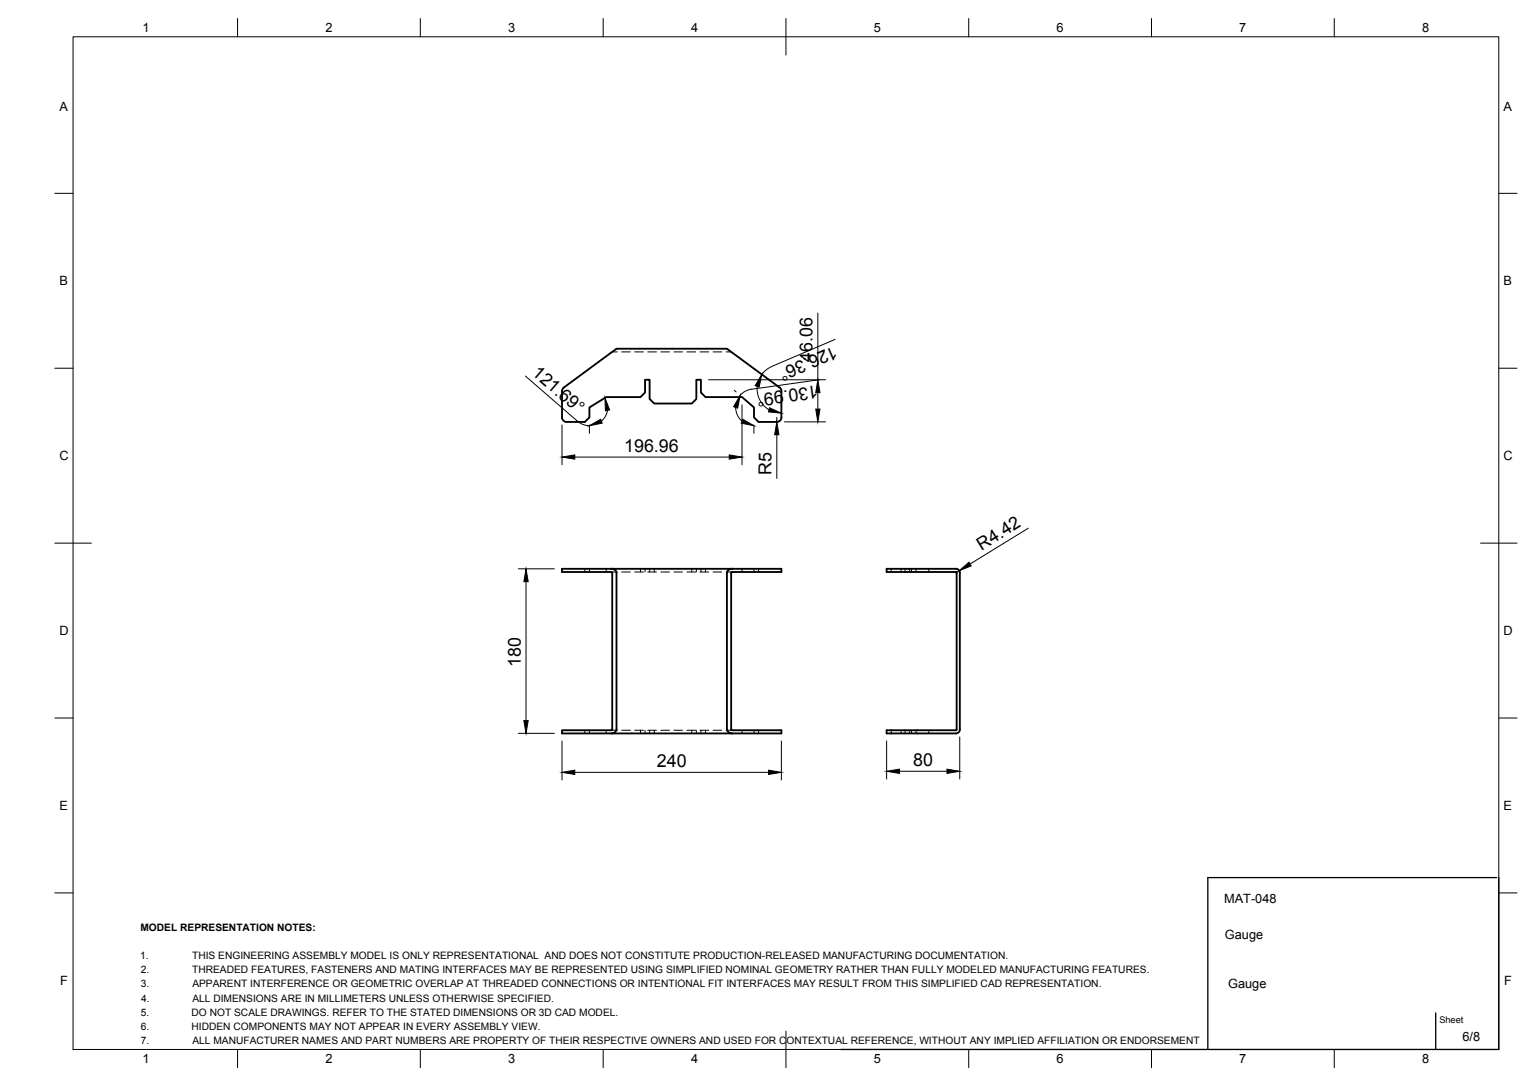
ISO-10303-21;
HEADER;
/* Generated by software containing ST-Developer
 * from STEP Tools, Inc. (www.steptools.com) 
 */

FILE_DESCRIPTION(
/* description */ ('STEP AP214'),
/* implementation_level */ '2;1');

FILE_NAME(
/* name */ 'Gauge.step',
/* time_stamp */ '2026-11-14T22:24:45-08:00',
/* author */ (''),
/* organization */ (''),
/* preprocessor_version */ 'ST-DEVELOPER v20.2',
/* originating_system */ 'Autodesk Translation Framework v15.17.0.0',
/* authorisation */ '');

FILE_SCHEMA (('AUTOMOTIVE_DESIGN { 1 0 10303 214 3 1 1 }'));
ENDSEC;

DATA;
#10=MECHANICAL_DESIGN_GEOMETRIC_PRESENTATION_REPRESENTATION('',(#125),#5599);
#113=SHAPE_REPRESENTATION_RELATIONSHIP('SRR','None',#5641,#119);
#119=ADVANCED_BREP_SHAPE_REPRESENTATION('',(#131),#5593);
#125=STYLED_ITEM('',(#5680),#131);
#131=MANIFOLD_SOLID_BREP('Body1',#3307);
#137=ELLIPSE('',#3398,7.45592114551632,4.41999999999987);
#138=ELLIPSE('',#3399,7.45592114551703,4.42000000000052);
#139=ELLIPSE('',#3402,7.45592114551723,4.42000000000049);
#140=ELLIPSE('',#3403,7.45592114551628,4.41999999999988);
#141=ELLIPSE('',#3416,1.68685998767419,1.00000000000061);
#142=ELLIPSE('',#3417,1.68685998767298,0.999999999999771);
#143=ELLIPSE('',#3420,1.68685998767017,0.999999999998458);
#144=ELLIPSE('',#3421,1.68685998767381,1.0000000000002);
#145=CYLINDRICAL_SURFACE('',#3397,4.42000000000001);
#146=CYLINDRICAL_SURFACE('',#3401,4.42);
#147=CYLINDRICAL_SURFACE('',#3415,1.);
#148=CYLINDRICAL_SURFACE('',#3419,1.);
#149=CYLINDRICAL_SURFACE('',#3464,5.);
#150=CYLINDRICAL_SURFACE('',#3465,5.);
#151=CYLINDRICAL_SURFACE('',#3466,5.);
#152=CYLINDRICAL_SURFACE('',#3467,5.);
#153=CYLINDRICAL_SURFACE('',#3468,5.);
#154=CYLINDRICAL_SURFACE('',#3469,5.);
#155=CYLINDRICAL_SURFACE('',#3470,5.);
#156=CYLINDRICAL_SURFACE('',#3471,5.);
#193=CIRCLE('',#3387,5.);
#194=CIRCLE('',#3388,5.);
#195=CIRCLE('',#3389,5.);
#196=CIRCLE('',#3390,5.);
#197=CIRCLE('',#3393,5.);
#198=CIRCLE('',#3394,5.);
#199=CIRCLE('',#3395,5.);
#200=CIRCLE('',#3396,5.);
#201=CIRCLE('',#3405,5.);
#202=CIRCLE('',#3406,5.);
#203=CIRCLE('',#3407,5.);
#204=CIRCLE('',#3408,5.);
#205=CIRCLE('',#3411,5.);
#206=CIRCLE('',#3412,5.);
#207=CIRCLE('',#3413,5.);
#208=CIRCLE('',#3414,5.);
#281=FACE_OUTER_BOUND('',#457,.T.);
#282=FACE_OUTER_BOUND('',#458,.T.);
#283=FACE_OUTER_BOUND('',#459,.T.);
#284=FACE_OUTER_BOUND('',#460,.T.);
#285=FACE_OUTER_BOUND('',#461,.T.);
#286=FACE_OUTER_BOUND('',#462,.T.);
#287=FACE_OUTER_BOUND('',#463,.T.);
#288=FACE_OUTER_BOUND('',#464,.T.);
#289=FACE_OUTER_BOUND('',#465,.T.);
#290=FACE_OUTER_BOUND('',#466,.T.);
#291=FACE_OUTER_BOUND('',#467,.T.);
#292=FACE_OUTER_BOUND('',#468,.T.);
#293=FACE_OUTER_BOUND('',#469,.T.);
#294=FACE_OUTER_BOUND('',#470,.T.);
#295=FACE_OUTER_BOUND('',#471,.T.);
#296=FACE_OUTER_BOUND('',#472,.T.);
#297=FACE_OUTER_BOUND('',#473,.T.);
#298=FACE_OUTER_BOUND('',#474,.T.);
#299=FACE_OUTER_BOUND('',#475,.T.);
#300=FACE_OUTER_BOUND('',#476,.T.);
#301=FACE_OUTER_BOUND('',#477,.T.);
#302=FACE_OUTER_BOUND('',#478,.T.);
#303=FACE_OUTER_BOUND('',#479,.T.);
#304=FACE_OUTER_BOUND('',#480,.T.);
#305=FACE_OUTER_BOUND('',#481,.T.);
#306=FACE_OUTER_BOUND('',#482,.T.);
#307=FACE_OUTER_BOUND('',#483,.T.);
#308=FACE_OUTER_BOUND('',#484,.T.);
#309=FACE_OUTER_BOUND('',#485,.T.);
#310=FACE_OUTER_BOUND('',#486,.T.);
#311=FACE_OUTER_BOUND('',#487,.T.);
#312=FACE_OUTER_BOUND('',#488,.T.);
#313=FACE_OUTER_BOUND('',#489,.T.);
#314=FACE_OUTER_BOUND('',#490,.T.);
#315=FACE_OUTER_BOUND('',#491,.T.);
#316=FACE_OUTER_BOUND('',#492,.T.);
#317=FACE_OUTER_BOUND('',#493,.T.);
#318=FACE_OUTER_BOUND('',#494,.T.);
#319=FACE_OUTER_BOUND('',#495,.T.);
#320=FACE_OUTER_BOUND('',#496,.T.);
#321=FACE_OUTER_BOUND('',#497,.T.);
#322=FACE_OUTER_BOUND('',#498,.T.);
#323=FACE_OUTER_BOUND('',#499,.T.);
#324=FACE_OUTER_BOUND('',#500,.T.);
#325=FACE_OUTER_BOUND('',#501,.T.);
#326=FACE_OUTER_BOUND('',#502,.T.);
#327=FACE_OUTER_BOUND('',#503,.T.);
#328=FACE_OUTER_BOUND('',#504,.T.);
#329=FACE_OUTER_BOUND('',#505,.T.);
#330=FACE_OUTER_BOUND('',#506,.T.);
#331=FACE_OUTER_BOUND('',#507,.T.);
#332=FACE_OUTER_BOUND('',#508,.T.);
#333=FACE_OUTER_BOUND('',#509,.T.);
#334=FACE_OUTER_BOUND('',#510,.T.);
#335=FACE_OUTER_BOUND('',#511,.T.);
#336=FACE_OUTER_BOUND('',#512,.T.);
#337=FACE_OUTER_BOUND('',#513,.T.);
#338=FACE_OUTER_BOUND('',#514,.T.);
#339=FACE_OUTER_BOUND('',#515,.T.);
#340=FACE_OUTER_BOUND('',#516,.T.);
#341=FACE_OUTER_BOUND('',#517,.T.);
#342=FACE_OUTER_BOUND('',#518,.T.);
#343=FACE_OUTER_BOUND('',#519,.T.);
#344=FACE_OUTER_BOUND('',#520,.T.);
#345=FACE_OUTER_BOUND('',#521,.T.);
#346=FACE_OUTER_BOUND('',#522,.T.);
#457=EDGE_LOOP('',(#2099,#2100,#2101,#2102));
#458=EDGE_LOOP('',(#2103,#2104,#2105,#2106));
#459=EDGE_LOOP('',(#2107,#2108,#2109,#2110));
#460=EDGE_LOOP('',(#2111,#2112,#2113,#2114));
#461=EDGE_LOOP('',(#2115,#2116,#2117,#2118,#2119,#2120,#2121,#2122,#2123,
#2124,#2125,#2126,#2127,#2128,#2129,#2130,#2131,#2132,#2133,#2134,#2135,
#2136,#2137,#2138,#2139,#2140,#2141,#2142,#2143,#2144));
#462=EDGE_LOOP('',(#2145,#2146,#2147,#2148));
#463=EDGE_LOOP('',(#2149,#2150,#2151,#2152,#2153,#2154,#2155,#2156,#2157,
#2158,#2159,#2160,#2161,#2162,#2163,#2164,#2165,#2166,#2167,#2168,#2169,
#2170,#2171,#2172,#2173,#2174,#2175,#2176,#2177,#2178));
#464=EDGE_LOOP('',(#2179,#2180,#2181,#2182));
#465=EDGE_LOOP('',(#2183,#2184,#2185,#2186));
#466=EDGE_LOOP('',(#2187,#2188,#2189,#2190));
#467=EDGE_LOOP('',(#2191,#2192,#2193,#2194,#2195,#2196,#2197,#2198,#2199,
#2200,#2201,#2202,#2203,#2204,#2205,#2206,#2207,#2208,#2209,#2210,#2211,
#2212,#2213,#2214,#2215,#2216,#2217,#2218,#2219,#2220));
#468=EDGE_LOOP('',(#2221,#2222,#2223,#2224));
#469=EDGE_LOOP('',(#2225,#2226,#2227,#2228,#2229,#2230,#2231,#2232,#2233,
#2234,#2235,#2236,#2237,#2238,#2239,#2240,#2241,#2242,#2243,#2244,#2245,
#2246,#2247,#2248,#2249,#2250,#2251,#2252,#2253,#2254));
#470=EDGE_LOOP('',(#2255,#2256,#2257,#2258));
#471=EDGE_LOOP('',(#2259,#2260,#2261,#2262));
#472=EDGE_LOOP('',(#2263,#2264,#2265,#2266));
#473=EDGE_LOOP('',(#2267,#2268,#2269,#2270));
#474=EDGE_LOOP('',(#2271,#2272,#2273,#2274));
#475=EDGE_LOOP('',(#2275,#2276,#2277,#2278,#2279,#2280,#2281,#2282,#2283,
#2284,#2285,#2286));
#476=EDGE_LOOP('',(#2287,#2288,#2289,#2290,#2291,#2292,#2293,#2294,#2295,
#2296,#2297,#2298));
#477=EDGE_LOOP('',(#2299,#2300,#2301,#2302));
#478=EDGE_LOOP('',(#2303,#2304,#2305,#2306));
#479=EDGE_LOOP('',(#2307,#2308,#2309,#2310));
#480=EDGE_LOOP('',(#2311,#2312,#2313,#2314));
#481=EDGE_LOOP('',(#2315,#2316,#2317,#2318));
#482=EDGE_LOOP('',(#2319,#2320,#2321,#2322));
#483=EDGE_LOOP('',(#2323,#2324,#2325,#2326));
#484=EDGE_LOOP('',(#2327,#2328,#2329,#2330));
#485=EDGE_LOOP('',(#2331,#2332,#2333,#2334));
#486=EDGE_LOOP('',(#2335,#2336,#2337,#2338));
#487=EDGE_LOOP('',(#2339,#2340,#2341,#2342));
#488=EDGE_LOOP('',(#2343,#2344,#2345,#2346));
#489=EDGE_LOOP('',(#2347,#2348,#2349,#2350));
#490=EDGE_LOOP('',(#2351,#2352,#2353,#2354));
#491=EDGE_LOOP('',(#2355,#2356,#2357,#2358));
#492=EDGE_LOOP('',(#2359,#2360,#2361,#2362));
#493=EDGE_LOOP('',(#2363,#2364,#2365,#2366));
#494=EDGE_LOOP('',(#2367,#2368,#2369,#2370));
#495=EDGE_LOOP('',(#2371,#2372,#2373,#2374));
#496=EDGE_LOOP('',(#2375,#2376,#2377,#2378));
#497=EDGE_LOOP('',(#2379,#2380,#2381,#2382));
#498=EDGE_LOOP('',(#2383,#2384,#2385,#2386));
#499=EDGE_LOOP('',(#2387,#2388,#2389,#2390));
#500=EDGE_LOOP('',(#2391,#2392,#2393,#2394));
#501=EDGE_LOOP('',(#2395,#2396,#2397,#2398));
#502=EDGE_LOOP('',(#2399,#2400,#2401,#2402));
#503=EDGE_LOOP('',(#2403,#2404,#2405,#2406));
#504=EDGE_LOOP('',(#2407,#2408,#2409,#2410));
#505=EDGE_LOOP('',(#2411,#2412,#2413,#2414));
#506=EDGE_LOOP('',(#2415,#2416,#2417,#2418));
#507=EDGE_LOOP('',(#2419,#2420,#2421,#2422));
#508=EDGE_LOOP('',(#2423,#2424,#2425,#2426));
#509=EDGE_LOOP('',(#2427,#2428,#2429,#2430));
#510=EDGE_LOOP('',(#2431,#2432,#2433,#2434));
#511=EDGE_LOOP('',(#2435,#2436,#2437,#2438));
#512=EDGE_LOOP('',(#2439,#2440,#2441,#2442));
#513=EDGE_LOOP('',(#2443,#2444,#2445,#2446));
#514=EDGE_LOOP('',(#2447,#2448,#2449,#2450));
#515=EDGE_LOOP('',(#2451,#2452,#2453,#2454));
#516=EDGE_LOOP('',(#2455,#2456,#2457,#2458));
#517=EDGE_LOOP('',(#2459,#2460,#2461,#2462));
#518=EDGE_LOOP('',(#2463,#2464,#2465,#2466));
#519=EDGE_LOOP('',(#2467,#2468,#2469,#2470));
#520=EDGE_LOOP('',(#2471,#2472,#2473,#2474));
#521=EDGE_LOOP('',(#2475,#2476,#2477,#2478));
#522=EDGE_LOOP('',(#2479,#2480,#2481,#2482));
#647=LINE('',#4644,#1003);
#648=LINE('',#4646,#1004);
#649=LINE('',#4648,#1005);
#650=LINE('',#4649,#1006);
#651=LINE('',#4653,#1007);
#652=LINE('',#4655,#1008);
#653=LINE('',#4657,#1009);
#654=LINE('',#4658,#1010);
#655=LINE('',#4662,#1011);
#656=LINE('',#4664,#1012);
#657=LINE('',#4666,#1013);
#658=LINE('',#4667,#1014);
#659=LINE('',#4671,#1015);
#660=LINE('',#4673,#1016);
#661=LINE('',#4675,#1017);
#662=LINE('',#4676,#1018);
#663=LINE('',#4680,#1019);
#664=LINE('',#4684,#1020);
#665=LINE('',#4686,#1021);
#666=LINE('',#4688,#1022);
#667=LINE('',#4690,#1023);
#668=LINE('',#4692,#1024);
#669=LINE('',#4694,#1025);
#670=LINE('',#4696,#1026);
#671=LINE('',#4698,#1027);
#672=LINE('',#4700,#1028);
#673=LINE('',#4702,#1029);
#674=LINE('',#4704,#1030);
#675=LINE('',#4706,#1031);
#676=LINE('',#4708,#1032);
#677=LINE('',#4710,#1033);
#678=LINE('',#4712,#1034);
#679=LINE('',#4714,#1035);
#680=LINE('',#4716,#1036);
#681=LINE('',#4718,#1037);
#682=LINE('',#4720,#1038);
#683=LINE('',#4721,#1039);
#684=LINE('',#4726,#1040);
#685=LINE('',#4728,#1041);
#686=LINE('',#4730,#1042);
#687=LINE('',#4734,#1043);
#688=LINE('',#4736,#1044);
#689=LINE('',#4737,#1045);
#690=LINE('',#4742,#1046);
#691=LINE('',#4746,#1047);
#692=LINE('',#4748,#1048);
#693=LINE('',#4750,#1049);
#694=LINE('',#4754,#1050);
#695=LINE('',#4756,#1051);
#696=LINE('',#4758,#1052);
#697=LINE('',#4760,#1053);
#698=LINE('',#4762,#1054);
#699=LINE('',#4764,#1055);
#700=LINE('',#4766,#1056);
#701=LINE('',#4768,#1057);
#702=LINE('',#4770,#1058);
#703=LINE('',#4772,#1059);
#704=LINE('',#4774,#1060);
#705=LINE('',#4776,#1061);
#706=LINE('',#4778,#1062);
#707=LINE('',#4780,#1063);
#708=LINE('',#4782,#1064);
#709=LINE('',#4784,#1065);
#710=LINE('',#4786,#1066);
#711=LINE('',#4788,#1067);
#712=LINE('',#4789,#1068);
#713=LINE('',#4795,#1069);
#714=LINE('',#4798,#1070);
#715=LINE('',#4800,#1071);
#716=LINE('',#4801,#1072);
#717=LINE('',#4807,#1073);
#718=LINE('',#4812,#1074);
#719=LINE('',#4814,#1075);
#720=LINE('',#4816,#1076);
#721=LINE('',#4818,#1077);
#722=LINE('',#4820,#1078);
#723=LINE('',#4822,#1079);
#724=LINE('',#4824,#1080);
#725=LINE('',#4826,#1081);
#726=LINE('',#4828,#1082);
#727=LINE('',#4830,#1083);
#728=LINE('',#4832,#1084);
#729=LINE('',#4834,#1085);
#730=LINE('',#4836,#1086);
#731=LINE('',#4838,#1087);
#732=LINE('',#4840,#1088);
#733=LINE('',#4842,#1089);
#734=LINE('',#4844,#1090);
#735=LINE('',#4846,#1091);
#736=LINE('',#4848,#1092);
#737=LINE('',#4849,#1093);
#738=LINE('',#4853,#1094);
#739=LINE('',#4856,#1095);
#740=LINE('',#4858,#1096);
#741=LINE('',#4862,#1097);
#742=LINE('',#4864,#1098);
#743=LINE('',#4865,#1099);
#744=LINE('',#4871,#1100);
#745=LINE('',#4873,#1101);
#746=LINE('',#4875,#1102);
#747=LINE('',#4879,#1103);
#748=LINE('',#4882,#1104);
#749=LINE('',#4884,#1105);
#750=LINE('',#4886,#1106);
#751=LINE('',#4888,#1107);
#752=LINE('',#4890,#1108);
#753=LINE('',#4892,#1109);
#754=LINE('',#4894,#1110);
#755=LINE('',#4896,#1111);
#756=LINE('',#4898,#1112);
#757=LINE('',#4900,#1113);
#758=LINE('',#4902,#1114);
#759=LINE('',#4904,#1115);
#760=LINE('',#4906,#1116);
#761=LINE('',#4908,#1117);
#762=LINE('',#4910,#1118);
#763=LINE('',#4912,#1119);
#764=LINE('',#4914,#1120);
#765=LINE('',#4916,#1121);
#766=LINE('',#4917,#1122);
#767=LINE('',#4921,#1123);
#768=LINE('',#4927,#1124);
#769=LINE('',#4928,#1125);
#770=LINE('',#4929,#1126);
#771=LINE('',#4934,#1127);
#772=LINE('',#4935,#1128);
#773=LINE('',#4937,#1129);
#774=LINE('',#4938,#1130);
#775=LINE('',#4940,#1131);
#776=LINE('',#4941,#1132);
#777=LINE('',#4943,#1133);
#778=LINE('',#4944,#1134);
#779=LINE('',#4946,#1135);
#780=LINE('',#4947,#1136);
#781=LINE('',#4949,#1137);
#782=LINE('',#4950,#1138);
#783=LINE('',#4952,#1139);
#784=LINE('',#4954,#1140);
#785=LINE('',#4956,#1141);
#786=LINE('',#4957,#1142);
#787=LINE('',#4959,#1143);
#788=LINE('',#4961,#1144);
#789=LINE('',#4963,#1145);
#790=LINE('',#4964,#1146);
#791=LINE('',#4966,#1147);
#792=LINE('',#4967,#1148);
#793=LINE('',#4969,#1149);
#794=LINE('',#4971,#1150);
#795=LINE('',#4973,#1151);
#796=LINE('',#4974,#1152);
#797=LINE('',#4977,#1153);
#798=LINE('',#4978,#1154);
#799=LINE('',#4980,#1155);
#800=LINE('',#4982,#1156);
#801=LINE('',#4983,#1157);
#802=LINE('',#4985,#1158);
#803=LINE('',#4987,#1159);
#804=LINE('',#4989,#1160);
#805=LINE('',#4990,#1161);
#806=LINE('',#4992,#1162);
#807=LINE('',#4993,#1163);
#808=LINE('',#4995,#1164);
#809=LINE('',#4997,#1165);
#810=LINE('',#4999,#1166);
#811=LINE('',#5000,#1167);
#812=LINE('',#5002,#1168);
#813=LINE('',#5004,#1169);
#814=LINE('',#5006,#1170);
#1003=VECTOR('',#3687,1000.);
#1004=VECTOR('',#3688,1000.);
#1005=VECTOR('',#3689,1000.);
#1006=VECTOR('',#3690,1000.);
#1007=VECTOR('',#3693,1000.);
#1008=VECTOR('',#3694,1000.);
#1009=VECTOR('',#3695,1000.);
#1010=VECTOR('',#3696,1000.);
#1011=VECTOR('',#3699,1000.);
#1012=VECTOR('',#3700,1000.);
#1013=VECTOR('',#3701,1000.);
#1014=VECTOR('',#3702,1000.);
#1015=VECTOR('',#3705,1000.);
#1016=VECTOR('',#3706,1000.);
#1017=VECTOR('',#3707,1000.);
#1018=VECTOR('',#3708,1000.);
#1019=VECTOR('',#3711,1000.);
#1020=VECTOR('',#3714,1000.);
#1021=VECTOR('',#3715,1000.);
#1022=VECTOR('',#3716,1000.);
#1023=VECTOR('',#3717,1000.);
#1024=VECTOR('',#3718,1000.);
#1025=VECTOR('',#3719,1000.);
#1026=VECTOR('',#3720,1000.);
#1027=VECTOR('',#3721,1000.);
#1028=VECTOR('',#3722,1000.);
#1029=VECTOR('',#3723,1000.);
#1030=VECTOR('',#3724,1000.);
#1031=VECTOR('',#3725,1000.);
#1032=VECTOR('',#3726,1000.);
#1033=VECTOR('',#3727,1000.);
#1034=VECTOR('',#3728,1000.);
#1035=VECTOR('',#3729,1000.);
#1036=VECTOR('',#3730,1000.);
#1037=VECTOR('',#3731,1000.);
#1038=VECTOR('',#3732,1000.);
#1039=VECTOR('',#3733,1000.);
#1040=VECTOR('',#3738,1000.);
#1041=VECTOR('',#3739,1000.);
#1042=VECTOR('',#3740,1000.);
#1043=VECTOR('',#3745,1000.);
#1044=VECTOR('',#3746,1000.);
#1045=VECTOR('',#3747,1000.);
#1046=VECTOR('',#3752,1000.);
#1047=VECTOR('',#3755,1000.);
#1048=VECTOR('',#3756,1000.);
#1049=VECTOR('',#3757,1000.);
#1050=VECTOR('',#3762,1000.);
#1051=VECTOR('',#3763,1000.);
#1052=VECTOR('',#3764,1000.);
#1053=VECTOR('',#3765,1000.);
#1054=VECTOR('',#3766,1000.);
#1055=VECTOR('',#3767,1000.);
#1056=VECTOR('',#3768,1000.);
#1057=VECTOR('',#3769,1000.);
#1058=VECTOR('',#3770,1000.);
#1059=VECTOR('',#3771,1000.);
#1060=VECTOR('',#3772,1000.);
#1061=VECTOR('',#3773,1000.);
#1062=VECTOR('',#3774,1000.);
#1063=VECTOR('',#3775,1000.);
#1064=VECTOR('',#3776,1000.);
#1065=VECTOR('',#3777,1000.);
#1066=VECTOR('',#3778,1000.);
#1067=VECTOR('',#3779,1000.);
#1068=VECTOR('',#3780,1000.);
#1069=VECTOR('',#3787,1000.);
#1070=VECTOR('',#3790,1000.);
#1071=VECTOR('',#3791,1000.);
#1072=VECTOR('',#3792,1000.);
#1073=VECTOR('',#3799,1000.);
#1074=VECTOR('',#3804,1000.);
#1075=VECTOR('',#3805,1000.);
#1076=VECTOR('',#3806,1000.);
#1077=VECTOR('',#3807,1000.);
#1078=VECTOR('',#3808,1000.);
#1079=VECTOR('',#3809,1000.);
#1080=VECTOR('',#3810,1000.);
#1081=VECTOR('',#3811,1000.);
#1082=VECTOR('',#3812,1000.);
#1083=VECTOR('',#3813,1000.);
#1084=VECTOR('',#3814,1000.);
#1085=VECTOR('',#3815,1000.);
#1086=VECTOR('',#3816,1000.);
#1087=VECTOR('',#3817,1000.);
#1088=VECTOR('',#3818,1000.);
#1089=VECTOR('',#3819,1000.);
#1090=VECTOR('',#3820,1000.);
#1091=VECTOR('',#3821,1000.);
#1092=VECTOR('',#3822,1000.);
#1093=VECTOR('',#3823,1000.);
#1094=VECTOR('',#3826,1000.);
#1095=VECTOR('',#3829,1000.);
#1096=VECTOR('',#3830,1000.);
#1097=VECTOR('',#3835,1000.);
#1098=VECTOR('',#3836,1000.);
#1099=VECTOR('',#3837,1000.);
#1100=VECTOR('',#3844,1000.);
#1101=VECTOR('',#3845,1000.);
#1102=VECTOR('',#3846,1000.);
#1103=VECTOR('',#3849,1000.);
#1104=VECTOR('',#3852,1000.);
#1105=VECTOR('',#3853,1000.);
#1106=VECTOR('',#3854,1000.);
#1107=VECTOR('',#3855,1000.);
#1108=VECTOR('',#3856,1000.);
#1109=VECTOR('',#3857,1000.);
#1110=VECTOR('',#3858,1000.);
#1111=VECTOR('',#3859,1000.);
#1112=VECTOR('',#3860,1000.);
#1113=VECTOR('',#3861,1000.);
#1114=VECTOR('',#3862,1000.);
#1115=VECTOR('',#3863,1000.);
#1116=VECTOR('',#3864,1000.);
#1117=VECTOR('',#3865,1000.);
#1118=VECTOR('',#3866,1000.);
#1119=VECTOR('',#3867,1000.);
#1120=VECTOR('',#3868,1000.);
#1121=VECTOR('',#3869,1000.);
#1122=VECTOR('',#3870,1000.);
#1123=VECTOR('',#3873,1000.);
#1124=VECTOR('',#3880,1000.);
#1125=VECTOR('',#3881,1000.);
#1126=VECTOR('',#3882,1000.);
#1127=VECTOR('',#3891,1000.);
#1128=VECTOR('',#3892,1000.);
#1129=VECTOR('',#3895,1000.);
#1130=VECTOR('',#3896,1000.);
#1131=VECTOR('',#3899,1000.);
#1132=VECTOR('',#3900,1000.);
#1133=VECTOR('',#3903,1000.);
#1134=VECTOR('',#3904,1000.);
#1135=VECTOR('',#3907,1000.);
#1136=VECTOR('',#3908,1000.);
#1137=VECTOR('',#3911,1000.);
#1138=VECTOR('',#3912,1000.);
#1139=VECTOR('',#3915,1000.);
#1140=VECTOR('',#3918,1000.);
#1141=VECTOR('',#3921,1000.);
#1142=VECTOR('',#3922,1000.);
#1143=VECTOR('',#3925,1000.);
#1144=VECTOR('',#3928,1000.);
#1145=VECTOR('',#3931,1000.);
#1146=VECTOR('',#3932,1000.);
#1147=VECTOR('',#3935,1000.);
#1148=VECTOR('',#3936,1000.);
#1149=VECTOR('',#3939,1000.);
#1150=VECTOR('',#3942,1000.);
#1151=VECTOR('',#3945,1000.);
#1152=VECTOR('',#3946,1000.);
#1153=VECTOR('',#3951,1000.);
#1154=VECTOR('',#3952,1000.);
#1155=VECTOR('',#3955,1000.);
#1156=VECTOR('',#3958,1000.);
#1157=VECTOR('',#3959,1000.);
#1158=VECTOR('',#3962,1000.);
#1159=VECTOR('',#3965,1000.);
#1160=VECTOR('',#3968,1000.);
#1161=VECTOR('',#3969,1000.);
#1162=VECTOR('',#3972,1000.);
#1163=VECTOR('',#3973,1000.);
#1164=VECTOR('',#3976,1000.);
#1165=VECTOR('',#3979,1000.);
#1166=VECTOR('',#3982,1000.);
#1167=VECTOR('',#3983,1000.);
#1168=VECTOR('',#3986,1000.);
#1169=VECTOR('',#3989,1000.);
#1170=VECTOR('',#3992,1000.);
#1359=VERTEX_POINT('',#4642);
#1360=VERTEX_POINT('',#4643);
#1361=VERTEX_POINT('',#4645);
#1362=VERTEX_POINT('',#4647);
#1363=VERTEX_POINT('',#4651);
#1364=VERTEX_POINT('',#4652);
#1365=VERTEX_POINT('',#4654);
#1366=VERTEX_POINT('',#4656);
#1367=VERTEX_POINT('',#4660);
#1368=VERTEX_POINT('',#4661);
#1369=VERTEX_POINT('',#4663);
#1370=VERTEX_POINT('',#4665);
#1371=VERTEX_POINT('',#4669);
#1372=VERTEX_POINT('',#4670);
#1373=VERTEX_POINT('',#4672);
#1374=VERTEX_POINT('',#4674);
#1375=VERTEX_POINT('',#4678);
#1376=VERTEX_POINT('',#4679);
#1377=VERTEX_POINT('',#4681);
#1378=VERTEX_POINT('',#4683);
#1379=VERTEX_POINT('',#4685);
#1380=VERTEX_POINT('',#4687);
#1381=VERTEX_POINT('',#4689);
#1382=VERTEX_POINT('',#4691);
#1383=VERTEX_POINT('',#4693);
#1384=VERTEX_POINT('',#4695);
#1385=VERTEX_POINT('',#4697);
#1386=VERTEX_POINT('',#4699);
#1387=VERTEX_POINT('',#4701);
#1388=VERTEX_POINT('',#4703);
#1389=VERTEX_POINT('',#4705);
#1390=VERTEX_POINT('',#4707);
#1391=VERTEX_POINT('',#4709);
#1392=VERTEX_POINT('',#4711);
#1393=VERTEX_POINT('',#4713);
#1394=VERTEX_POINT('',#4715);
#1395=VERTEX_POINT('',#4717);
#1396=VERTEX_POINT('',#4719);
#1397=VERTEX_POINT('',#4723);
#1398=VERTEX_POINT('',#4725);
#1399=VERTEX_POINT('',#4727);
#1400=VERTEX_POINT('',#4729);
#1401=VERTEX_POINT('',#4733);
#1402=VERTEX_POINT('',#4735);
#1403=VERTEX_POINT('',#4739);
#1404=VERTEX_POINT('',#4741);
#1405=VERTEX_POINT('',#4743);
#1406=VERTEX_POINT('',#4745);
#1407=VERTEX_POINT('',#4747);
#1408=VERTEX_POINT('',#4749);
#1409=VERTEX_POINT('',#4753);
#1410=VERTEX_POINT('',#4755);
#1411=VERTEX_POINT('',#4757);
#1412=VERTEX_POINT('',#4759);
#1413=VERTEX_POINT('',#4761);
#1414=VERTEX_POINT('',#4763);
#1415=VERTEX_POINT('',#4765);
#1416=VERTEX_POINT('',#4767);
#1417=VERTEX_POINT('',#4769);
#1418=VERTEX_POINT('',#4771);
#1419=VERTEX_POINT('',#4773);
#1420=VERTEX_POINT('',#4775);
#1421=VERTEX_POINT('',#4777);
#1422=VERTEX_POINT('',#4779);
#1423=VERTEX_POINT('',#4781);
#1424=VERTEX_POINT('',#4783);
#1425=VERTEX_POINT('',#4785);
#1426=VERTEX_POINT('',#4787);
#1427=VERTEX_POINT('',#4791);
#1428=VERTEX_POINT('',#4793);
#1429=VERTEX_POINT('',#4797);
#1430=VERTEX_POINT('',#4799);
#1431=VERTEX_POINT('',#4803);
#1432=VERTEX_POINT('',#4805);
#1433=VERTEX_POINT('',#4809);
#1434=VERTEX_POINT('',#4811);
#1435=VERTEX_POINT('',#4813);
#1436=VERTEX_POINT('',#4815);
#1437=VERTEX_POINT('',#4817);
#1438=VERTEX_POINT('',#4819);
#1439=VERTEX_POINT('',#4821);
#1440=VERTEX_POINT('',#4823);
#1441=VERTEX_POINT('',#4825);
#1442=VERTEX_POINT('',#4827);
#1443=VERTEX_POINT('',#4829);
#1444=VERTEX_POINT('',#4831);
#1445=VERTEX_POINT('',#4833);
#1446=VERTEX_POINT('',#4835);
#1447=VERTEX_POINT('',#4837);
#1448=VERTEX_POINT('',#4839);
#1449=VERTEX_POINT('',#4841);
#1450=VERTEX_POINT('',#4843);
#1451=VERTEX_POINT('',#4845);
#1452=VERTEX_POINT('',#4847);
#1453=VERTEX_POINT('',#4850);
#1454=VERTEX_POINT('',#4852);
#1455=VERTEX_POINT('',#4854);
#1456=VERTEX_POINT('',#4857);
#1457=VERTEX_POINT('',#4861);
#1458=VERTEX_POINT('',#4863);
#1459=VERTEX_POINT('',#4868);
#1460=VERTEX_POINT('',#4870);
#1461=VERTEX_POINT('',#4872);
#1462=VERTEX_POINT('',#4874);
#1463=VERTEX_POINT('',#4876);
#1464=VERTEX_POINT('',#4878);
#1465=VERTEX_POINT('',#4881);
#1466=VERTEX_POINT('',#4883);
#1467=VERTEX_POINT('',#4885);
#1468=VERTEX_POINT('',#4887);
#1469=VERTEX_POINT('',#4889);
#1470=VERTEX_POINT('',#4891);
#1471=VERTEX_POINT('',#4893);
#1472=VERTEX_POINT('',#4895);
#1473=VERTEX_POINT('',#4897);
#1474=VERTEX_POINT('',#4899);
#1475=VERTEX_POINT('',#4901);
#1476=VERTEX_POINT('',#4903);
#1477=VERTEX_POINT('',#4905);
#1478=VERTEX_POINT('',#4907);
#1479=VERTEX_POINT('',#4909);
#1480=VERTEX_POINT('',#4911);
#1481=VERTEX_POINT('',#4913);
#1482=VERTEX_POINT('',#4915);
#1483=VERTEX_POINT('',#4919);
#1484=VERTEX_POINT('',#4920);
#1485=VERTEX_POINT('',#4925);
#1486=VERTEX_POINT('',#4926);
#1647=EDGE_CURVE('',#1359,#1360,#647,.T.);
#1648=EDGE_CURVE('',#1359,#1361,#648,.T.);
#1649=EDGE_CURVE('',#1361,#1362,#649,.T.);
#1650=EDGE_CURVE('',#1362,#1360,#650,.T.);
#1651=EDGE_CURVE('',#1363,#1364,#651,.T.);
#1652=EDGE_CURVE('',#1363,#1365,#652,.T.);
#1653=EDGE_CURVE('',#1365,#1366,#653,.T.);
#1654=EDGE_CURVE('',#1366,#1364,#654,.T.);
#1655=EDGE_CURVE('',#1367,#1368,#655,.T.);
#1656=EDGE_CURVE('',#1367,#1369,#656,.T.);
#1657=EDGE_CURVE('',#1369,#1370,#657,.T.);
#1658=EDGE_CURVE('',#1370,#1368,#658,.T.);
#1659=EDGE_CURVE('',#1371,#1372,#659,.T.);
#1660=EDGE_CURVE('',#1372,#1373,#660,.T.);
#1661=EDGE_CURVE('',#1374,#1373,#661,.T.);
#1662=EDGE_CURVE('',#1374,#1371,#662,.T.);
#1663=EDGE_CURVE('',#1375,#1376,#663,.T.);
#1664=EDGE_CURVE('',#1376,#1377,#193,.T.);
#1665=EDGE_CURVE('',#1378,#1377,#664,.T.);
#1666=EDGE_CURVE('',#1378,#1379,#665,.T.);
#1667=EDGE_CURVE('',#1379,#1380,#666,.T.);
#1668=EDGE_CURVE('',#1380,#1381,#667,.T.);
#1669=EDGE_CURVE('',#1381,#1382,#668,.T.);
#1670=EDGE_CURVE('',#1382,#1383,#669,.T.);
#1671=EDGE_CURVE('',#1383,#1384,#670,.T.);
#1672=EDGE_CURVE('',#1384,#1385,#671,.T.);
#1673=EDGE_CURVE('',#1385,#1386,#672,.T.);
#1674=EDGE_CURVE('',#1386,#1387,#673,.T.);
#1675=EDGE_CURVE('',#1387,#1388,#674,.T.);
#1676=EDGE_CURVE('',#1388,#1389,#675,.T.);
#1677=EDGE_CURVE('',#1389,#1390,#676,.T.);
#1678=EDGE_CURVE('',#1390,#1391,#677,.T.);
#1679=EDGE_CURVE('',#1391,#1392,#678,.T.);
#1680=EDGE_CURVE('',#1392,#1393,#679,.T.);
#1681=EDGE_CURVE('',#1393,#1394,#680,.T.);
#1682=EDGE_CURVE('',#1394,#1395,#681,.T.);
#1683=EDGE_CURVE('',#1395,#1396,#682,.T.);
#1684=EDGE_CURVE('',#1396,#1362,#683,.T.);
#1685=EDGE_CURVE('',#1361,#1372,#194,.T.);
#1686=EDGE_CURVE('',#1371,#1397,#195,.T.);
#1687=EDGE_CURVE('',#1397,#1398,#684,.T.);
#1688=EDGE_CURVE('',#1398,#1399,#685,.T.);
#1689=EDGE_CURVE('',#1399,#1400,#686,.T.);
#1690=EDGE_CURVE('',#1400,#1375,#196,.T.);
#1691=EDGE_CURVE('',#1377,#1401,#687,.T.);
#1692=EDGE_CURVE('',#1402,#1401,#688,.T.);
#1693=EDGE_CURVE('',#1402,#1378,#689,.T.);
#1694=EDGE_CURVE('',#1401,#1403,#197,.T.);
#1695=EDGE_CURVE('',#1404,#1403,#690,.T.);
#1696=EDGE_CURVE('',#1404,#1405,#198,.T.);
#1697=EDGE_CURVE('',#1405,#1406,#691,.T.);
#1698=EDGE_CURVE('',#1407,#1406,#692,.T.);
#1699=EDGE_CURVE('',#1407,#1408,#693,.T.);
#1700=EDGE_CURVE('',#1408,#1374,#199,.T.);
#1701=EDGE_CURVE('',#1373,#1359,#200,.T.);
#1702=EDGE_CURVE('',#1360,#1409,#694,.T.);
#1703=EDGE_CURVE('',#1409,#1410,#695,.T.);
#1704=EDGE_CURVE('',#1410,#1411,#696,.T.);
#1705=EDGE_CURVE('',#1411,#1412,#697,.T.);
#1706=EDGE_CURVE('',#1412,#1413,#698,.T.);
#1707=EDGE_CURVE('',#1413,#1414,#699,.T.);
#1708=EDGE_CURVE('',#1414,#1415,#700,.T.);
#1709=EDGE_CURVE('',#1415,#1416,#701,.T.);
#1710=EDGE_CURVE('',#1416,#1417,#702,.T.);
#1711=EDGE_CURVE('',#1417,#1418,#703,.T.);
#1712=EDGE_CURVE('',#1418,#1419,#704,.T.);
#1713=EDGE_CURVE('',#1419,#1420,#705,.T.);
#1714=EDGE_CURVE('',#1420,#1421,#706,.T.);
#1715=EDGE_CURVE('',#1421,#1422,#707,.T.);
#1716=EDGE_CURVE('',#1422,#1423,#708,.T.);
#1717=EDGE_CURVE('',#1423,#1424,#709,.T.);
#1718=EDGE_CURVE('',#1424,#1425,#710,.T.);
#1719=EDGE_CURVE('',#1425,#1426,#711,.T.);
#1720=EDGE_CURVE('',#1426,#1402,#712,.T.);
#1721=EDGE_CURVE('',#1407,#1427,#137,.T.);
#1722=EDGE_CURVE('',#1428,#1406,#138,.T.);
#1723=EDGE_CURVE('',#1427,#1428,#713,.T.);
#1724=EDGE_CURVE('',#1427,#1429,#714,.T.);
#1725=EDGE_CURVE('',#1430,#1428,#715,.T.);
#1726=EDGE_CURVE('',#1429,#1430,#716,.T.);
#1727=EDGE_CURVE('',#1429,#1431,#139,.T.);
#1728=EDGE_CURVE('',#1432,#1430,#140,.T.);
#1729=EDGE_CURVE('',#1431,#1432,#717,.T.);
#1730=EDGE_CURVE('',#1369,#1433,#201,.T.);
#1731=EDGE_CURVE('',#1434,#1433,#718,.T.);
#1732=EDGE_CURVE('',#1434,#1435,#719,.T.);
#1733=EDGE_CURVE('',#1436,#1435,#720,.T.);
#1734=EDGE_CURVE('',#1437,#1436,#721,.T.);
#1735=EDGE_CURVE('',#1438,#1437,#722,.T.);
#1736=EDGE_CURVE('',#1438,#1439,#723,.T.);
#1737=EDGE_CURVE('',#1440,#1439,#724,.T.);
#1738=EDGE_CURVE('',#1441,#1440,#725,.T.);
#1739=EDGE_CURVE('',#1442,#1441,#726,.T.);
#1740=EDGE_CURVE('',#1442,#1443,#727,.T.);
#1741=EDGE_CURVE('',#1444,#1443,#728,.T.);
#1742=EDGE_CURVE('',#1444,#1445,#729,.T.);
#1743=EDGE_CURVE('',#1446,#1445,#730,.T.);
#1744=EDGE_CURVE('',#1447,#1446,#731,.T.);
#1745=EDGE_CURVE('',#1448,#1447,#732,.T.);
#1746=EDGE_CURVE('',#1448,#1449,#733,.T.);
#1747=EDGE_CURVE('',#1450,#1449,#734,.T.);
#1748=EDGE_CURVE('',#1451,#1450,#735,.T.);
#1749=EDGE_CURVE('',#1452,#1451,#736,.T.);
#1750=EDGE_CURVE('',#1452,#1366,#737,.T.);
#1751=EDGE_CURVE('',#1365,#1453,#202,.T.);
#1752=EDGE_CURVE('',#1453,#1454,#738,.T.);
#1753=EDGE_CURVE('',#1454,#1455,#203,.T.);
#1754=EDGE_CURVE('',#1431,#1455,#739,.T.);
#1755=EDGE_CURVE('',#1456,#1432,#740,.T.);
#1756=EDGE_CURVE('',#1456,#1370,#204,.T.);
#1757=EDGE_CURVE('',#1433,#1457,#741,.T.);
#1758=EDGE_CURVE('',#1458,#1457,#742,.T.);
#1759=EDGE_CURVE('',#1458,#1434,#743,.T.);
#1760=EDGE_CURVE('',#1457,#1367,#205,.T.);
#1761=EDGE_CURVE('',#1368,#1459,#206,.T.);
#1762=EDGE_CURVE('',#1459,#1460,#744,.T.);
#1763=EDGE_CURVE('',#1461,#1460,#745,.T.);
#1764=EDGE_CURVE('',#1461,#1462,#746,.T.);
#1765=EDGE_CURVE('',#1462,#1463,#207,.T.);
#1766=EDGE_CURVE('',#1464,#1463,#747,.T.);
#1767=EDGE_CURVE('',#1464,#1363,#208,.T.);
#1768=EDGE_CURVE('',#1364,#1465,#748,.T.);
#1769=EDGE_CURVE('',#1465,#1466,#749,.T.);
#1770=EDGE_CURVE('',#1466,#1467,#750,.T.);
#1771=EDGE_CURVE('',#1467,#1468,#751,.T.);
#1772=EDGE_CURVE('',#1468,#1469,#752,.T.);
#1773=EDGE_CURVE('',#1469,#1470,#753,.T.);
#1774=EDGE_CURVE('',#1470,#1471,#754,.T.);
#1775=EDGE_CURVE('',#1471,#1472,#755,.T.);
#1776=EDGE_CURVE('',#1472,#1473,#756,.T.);
#1777=EDGE_CURVE('',#1473,#1474,#757,.T.);
#1778=EDGE_CURVE('',#1474,#1475,#758,.T.);
#1779=EDGE_CURVE('',#1475,#1476,#759,.T.);
#1780=EDGE_CURVE('',#1476,#1477,#760,.T.);
#1781=EDGE_CURVE('',#1477,#1478,#761,.T.);
#1782=EDGE_CURVE('',#1478,#1479,#762,.T.);
#1783=EDGE_CURVE('',#1479,#1480,#763,.T.);
#1784=EDGE_CURVE('',#1480,#1481,#764,.T.);
#1785=EDGE_CURVE('',#1481,#1482,#765,.T.);
#1786=EDGE_CURVE('',#1482,#1458,#766,.T.);
#1787=EDGE_CURVE('',#1483,#1484,#767,.T.);
#1788=EDGE_CURVE('',#1483,#1461,#141,.T.);
#1789=EDGE_CURVE('',#1460,#1484,#142,.T.);
#1790=EDGE_CURVE('',#1485,#1486,#768,.T.);
#1791=EDGE_CURVE('',#1485,#1483,#769,.T.);
#1792=EDGE_CURVE('',#1484,#1486,#770,.T.);
#1793=EDGE_CURVE('',#1398,#1485,#143,.T.);
#1794=EDGE_CURVE('',#1486,#1399,#144,.T.);
#1795=EDGE_CURVE('',#1453,#1464,#771,.T.);
#1796=EDGE_CURVE('',#1463,#1454,#772,.T.);
#1797=EDGE_CURVE('',#1403,#1376,#773,.T.);
#1798=EDGE_CURVE('',#1375,#1404,#774,.T.);
#1799=EDGE_CURVE('',#1459,#1456,#775,.T.);
#1800=EDGE_CURVE('',#1405,#1400,#776,.T.);
#1801=EDGE_CURVE('',#1397,#1408,#777,.T.);
#1802=EDGE_CURVE('',#1455,#1462,#778,.T.);
#1803=EDGE_CURVE('',#1435,#1482,#779,.T.);
#1804=EDGE_CURVE('',#1481,#1436,#780,.T.);
#1805=EDGE_CURVE('',#1465,#1452,#781,.T.);
#1806=EDGE_CURVE('',#1466,#1451,#782,.T.);
#1807=EDGE_CURVE('',#1467,#1450,#783,.T.);
#1808=EDGE_CURVE('',#1449,#1468,#784,.T.);
#1809=EDGE_CURVE('',#1469,#1448,#785,.T.);
#1810=EDGE_CURVE('',#1470,#1447,#786,.T.);
#1811=EDGE_CURVE('',#1471,#1446,#787,.T.);
#1812=EDGE_CURVE('',#1445,#1472,#788,.T.);
#1813=EDGE_CURVE('',#1443,#1474,#789,.T.);
#1814=EDGE_CURVE('',#1473,#1444,#790,.T.);
#1815=EDGE_CURVE('',#1475,#1442,#791,.T.);
#1816=EDGE_CURVE('',#1476,#1441,#792,.T.);
#1817=EDGE_CURVE('',#1477,#1440,#793,.T.);
#1818=EDGE_CURVE('',#1439,#1478,#794,.T.);
#1819=EDGE_CURVE('',#1479,#1438,#795,.T.);
#1820=EDGE_CURVE('',#1480,#1437,#796,.T.);
#1821=EDGE_CURVE('',#1425,#1380,#797,.T.);
#1822=EDGE_CURVE('',#1424,#1381,#798,.T.);
#1823=EDGE_CURVE('',#1423,#1382,#799,.T.);
#1824=EDGE_CURVE('',#1383,#1422,#800,.T.);
#1825=EDGE_CURVE('',#1421,#1384,#801,.T.);
#1826=EDGE_CURVE('',#1420,#1385,#802,.T.);
#1827=EDGE_CURVE('',#1419,#1386,#803,.T.);
#1828=EDGE_CURVE('',#1387,#1418,#804,.T.);
#1829=EDGE_CURVE('',#1417,#1388,#805,.T.);
#1830=EDGE_CURVE('',#1389,#1416,#806,.T.);
#1831=EDGE_CURVE('',#1415,#1390,#807,.T.);
#1832=EDGE_CURVE('',#1414,#1391,#808,.T.);
#1833=EDGE_CURVE('',#1413,#1392,#809,.T.);
#1834=EDGE_CURVE('',#1393,#1412,#810,.T.);
#1835=EDGE_CURVE('',#1411,#1394,#811,.T.);
#1836=EDGE_CURVE('',#1410,#1395,#812,.T.);
#1837=EDGE_CURVE('',#1409,#1396,#813,.T.);
#1838=EDGE_CURVE('',#1379,#1426,#814,.T.);
#2099=ORIENTED_EDGE('',*,*,#1647,.F.);
#2100=ORIENTED_EDGE('',*,*,#1648,.T.);
#2101=ORIENTED_EDGE('',*,*,#1649,.T.);
#2102=ORIENTED_EDGE('',*,*,#1650,.T.);
#2103=ORIENTED_EDGE('',*,*,#1651,.F.);
#2104=ORIENTED_EDGE('',*,*,#1652,.T.);
#2105=ORIENTED_EDGE('',*,*,#1653,.T.);
#2106=ORIENTED_EDGE('',*,*,#1654,.T.);
#2107=ORIENTED_EDGE('',*,*,#1655,.F.);
#2108=ORIENTED_EDGE('',*,*,#1656,.T.);
#2109=ORIENTED_EDGE('',*,*,#1657,.T.);
#2110=ORIENTED_EDGE('',*,*,#1658,.T.);
#2111=ORIENTED_EDGE('',*,*,#1659,.T.);
#2112=ORIENTED_EDGE('',*,*,#1660,.T.);
#2113=ORIENTED_EDGE('',*,*,#1661,.F.);
#2114=ORIENTED_EDGE('',*,*,#1662,.T.);
#2115=ORIENTED_EDGE('',*,*,#1663,.T.);
#2116=ORIENTED_EDGE('',*,*,#1664,.T.);
#2117=ORIENTED_EDGE('',*,*,#1665,.F.);
#2118=ORIENTED_EDGE('',*,*,#1666,.T.);
#2119=ORIENTED_EDGE('',*,*,#1667,.T.);
#2120=ORIENTED_EDGE('',*,*,#1668,.T.);
#2121=ORIENTED_EDGE('',*,*,#1669,.T.);
#2122=ORIENTED_EDGE('',*,*,#1670,.T.);
#2123=ORIENTED_EDGE('',*,*,#1671,.T.);
#2124=ORIENTED_EDGE('',*,*,#1672,.T.);
#2125=ORIENTED_EDGE('',*,*,#1673,.T.);
#2126=ORIENTED_EDGE('',*,*,#1674,.T.);
#2127=ORIENTED_EDGE('',*,*,#1675,.T.);
#2128=ORIENTED_EDGE('',*,*,#1676,.T.);
#2129=ORIENTED_EDGE('',*,*,#1677,.T.);
#2130=ORIENTED_EDGE('',*,*,#1678,.T.);
#2131=ORIENTED_EDGE('',*,*,#1679,.T.);
#2132=ORIENTED_EDGE('',*,*,#1680,.T.);
#2133=ORIENTED_EDGE('',*,*,#1681,.T.);
#2134=ORIENTED_EDGE('',*,*,#1682,.T.);
#2135=ORIENTED_EDGE('',*,*,#1683,.T.);
#2136=ORIENTED_EDGE('',*,*,#1684,.T.);
#2137=ORIENTED_EDGE('',*,*,#1649,.F.);
#2138=ORIENTED_EDGE('',*,*,#1685,.T.);
#2139=ORIENTED_EDGE('',*,*,#1659,.F.);
#2140=ORIENTED_EDGE('',*,*,#1686,.T.);
#2141=ORIENTED_EDGE('',*,*,#1687,.T.);
#2142=ORIENTED_EDGE('',*,*,#1688,.T.);
#2143=ORIENTED_EDGE('',*,*,#1689,.T.);
#2144=ORIENTED_EDGE('',*,*,#1690,.T.);
#2145=ORIENTED_EDGE('',*,*,#1665,.T.);
#2146=ORIENTED_EDGE('',*,*,#1691,.T.);
#2147=ORIENTED_EDGE('',*,*,#1692,.F.);
#2148=ORIENTED_EDGE('',*,*,#1693,.T.);
#2149=ORIENTED_EDGE('',*,*,#1692,.T.);
#2150=ORIENTED_EDGE('',*,*,#1694,.T.);
#2151=ORIENTED_EDGE('',*,*,#1695,.F.);
#2152=ORIENTED_EDGE('',*,*,#1696,.T.);
#2153=ORIENTED_EDGE('',*,*,#1697,.T.);
#2154=ORIENTED_EDGE('',*,*,#1698,.F.);
#2155=ORIENTED_EDGE('',*,*,#1699,.T.);
#2156=ORIENTED_EDGE('',*,*,#1700,.T.);
#2157=ORIENTED_EDGE('',*,*,#1661,.T.);
#2158=ORIENTED_EDGE('',*,*,#1701,.T.);
#2159=ORIENTED_EDGE('',*,*,#1647,.T.);
#2160=ORIENTED_EDGE('',*,*,#1702,.T.);
#2161=ORIENTED_EDGE('',*,*,#1703,.T.);
#2162=ORIENTED_EDGE('',*,*,#1704,.T.);
#2163=ORIENTED_EDGE('',*,*,#1705,.T.);
#2164=ORIENTED_EDGE('',*,*,#1706,.T.);
#2165=ORIENTED_EDGE('',*,*,#1707,.T.);
#2166=ORIENTED_EDGE('',*,*,#1708,.T.);
#2167=ORIENTED_EDGE('',*,*,#1709,.T.);
#2168=ORIENTED_EDGE('',*,*,#1710,.T.);
#2169=ORIENTED_EDGE('',*,*,#1711,.T.);
#2170=ORIENTED_EDGE('',*,*,#1712,.T.);
#2171=ORIENTED_EDGE('',*,*,#1713,.T.);
#2172=ORIENTED_EDGE('',*,*,#1714,.T.);
#2173=ORIENTED_EDGE('',*,*,#1715,.T.);
#2174=ORIENTED_EDGE('',*,*,#1716,.T.);
#2175=ORIENTED_EDGE('',*,*,#1717,.T.);
#2176=ORIENTED_EDGE('',*,*,#1718,.T.);
#2177=ORIENTED_EDGE('',*,*,#1719,.T.);
#2178=ORIENTED_EDGE('',*,*,#1720,.T.);
#2179=ORIENTED_EDGE('',*,*,#1721,.F.);
#2180=ORIENTED_EDGE('',*,*,#1698,.T.);
#2181=ORIENTED_EDGE('',*,*,#1722,.F.);
#2182=ORIENTED_EDGE('',*,*,#1723,.F.);
#2183=ORIENTED_EDGE('',*,*,#1724,.F.);
#2184=ORIENTED_EDGE('',*,*,#1723,.T.);
#2185=ORIENTED_EDGE('',*,*,#1725,.F.);
#2186=ORIENTED_EDGE('',*,*,#1726,.F.);
#2187=ORIENTED_EDGE('',*,*,#1727,.F.);
#2188=ORIENTED_EDGE('',*,*,#1726,.T.);
#2189=ORIENTED_EDGE('',*,*,#1728,.F.);
#2190=ORIENTED_EDGE('',*,*,#1729,.F.);
#2191=ORIENTED_EDGE('',*,*,#1657,.F.);
#2192=ORIENTED_EDGE('',*,*,#1730,.T.);
#2193=ORIENTED_EDGE('',*,*,#1731,.F.);
#2194=ORIENTED_EDGE('',*,*,#1732,.T.);
#2195=ORIENTED_EDGE('',*,*,#1733,.F.);
#2196=ORIENTED_EDGE('',*,*,#1734,.F.);
#2197=ORIENTED_EDGE('',*,*,#1735,.F.);
#2198=ORIENTED_EDGE('',*,*,#1736,.T.);
#2199=ORIENTED_EDGE('',*,*,#1737,.F.);
#2200=ORIENTED_EDGE('',*,*,#1738,.F.);
#2201=ORIENTED_EDGE('',*,*,#1739,.F.);
#2202=ORIENTED_EDGE('',*,*,#1740,.T.);
#2203=ORIENTED_EDGE('',*,*,#1741,.F.);
#2204=ORIENTED_EDGE('',*,*,#1742,.T.);
#2205=ORIENTED_EDGE('',*,*,#1743,.F.);
#2206=ORIENTED_EDGE('',*,*,#1744,.F.);
#2207=ORIENTED_EDGE('',*,*,#1745,.F.);
#2208=ORIENTED_EDGE('',*,*,#1746,.T.);
#2209=ORIENTED_EDGE('',*,*,#1747,.F.);
#2210=ORIENTED_EDGE('',*,*,#1748,.F.);
#2211=ORIENTED_EDGE('',*,*,#1749,.F.);
#2212=ORIENTED_EDGE('',*,*,#1750,.T.);
#2213=ORIENTED_EDGE('',*,*,#1653,.F.);
#2214=ORIENTED_EDGE('',*,*,#1751,.T.);
#2215=ORIENTED_EDGE('',*,*,#1752,.T.);
#2216=ORIENTED_EDGE('',*,*,#1753,.T.);
#2217=ORIENTED_EDGE('',*,*,#1754,.F.);
#2218=ORIENTED_EDGE('',*,*,#1729,.T.);
#2219=ORIENTED_EDGE('',*,*,#1755,.F.);
#2220=ORIENTED_EDGE('',*,*,#1756,.T.);
#2221=ORIENTED_EDGE('',*,*,#1731,.T.);
#2222=ORIENTED_EDGE('',*,*,#1757,.T.);
#2223=ORIENTED_EDGE('',*,*,#1758,.F.);
#2224=ORIENTED_EDGE('',*,*,#1759,.T.);
#2225=ORIENTED_EDGE('',*,*,#1758,.T.);
#2226=ORIENTED_EDGE('',*,*,#1760,.T.);
#2227=ORIENTED_EDGE('',*,*,#1655,.T.);
#2228=ORIENTED_EDGE('',*,*,#1761,.T.);
#2229=ORIENTED_EDGE('',*,*,#1762,.T.);
#2230=ORIENTED_EDGE('',*,*,#1763,.F.);
#2231=ORIENTED_EDGE('',*,*,#1764,.T.);
#2232=ORIENTED_EDGE('',*,*,#1765,.T.);
#2233=ORIENTED_EDGE('',*,*,#1766,.F.);
#2234=ORIENTED_EDGE('',*,*,#1767,.T.);
#2235=ORIENTED_EDGE('',*,*,#1651,.T.);
#2236=ORIENTED_EDGE('',*,*,#1768,.T.);
#2237=ORIENTED_EDGE('',*,*,#1769,.T.);
#2238=ORIENTED_EDGE('',*,*,#1770,.T.);
#2239=ORIENTED_EDGE('',*,*,#1771,.T.);
#2240=ORIENTED_EDGE('',*,*,#1772,.T.);
#2241=ORIENTED_EDGE('',*,*,#1773,.T.);
#2242=ORIENTED_EDGE('',*,*,#1774,.T.);
#2243=ORIENTED_EDGE('',*,*,#1775,.T.);
#2244=ORIENTED_EDGE('',*,*,#1776,.T.);
#2245=ORIENTED_EDGE('',*,*,#1777,.T.);
#2246=ORIENTED_EDGE('',*,*,#1778,.T.);
#2247=ORIENTED_EDGE('',*,*,#1779,.T.);
#2248=ORIENTED_EDGE('',*,*,#1780,.T.);
#2249=ORIENTED_EDGE('',*,*,#1781,.T.);
#2250=ORIENTED_EDGE('',*,*,#1782,.T.);
#2251=ORIENTED_EDGE('',*,*,#1783,.T.);
#2252=ORIENTED_EDGE('',*,*,#1784,.T.);
#2253=ORIENTED_EDGE('',*,*,#1785,.T.);
#2254=ORIENTED_EDGE('',*,*,#1786,.T.);
#2255=ORIENTED_EDGE('',*,*,#1787,.F.);
#2256=ORIENTED_EDGE('',*,*,#1788,.T.);
#2257=ORIENTED_EDGE('',*,*,#1763,.T.);
#2258=ORIENTED_EDGE('',*,*,#1789,.T.);
#2259=ORIENTED_EDGE('',*,*,#1790,.F.);
#2260=ORIENTED_EDGE('',*,*,#1791,.T.);
#2261=ORIENTED_EDGE('',*,*,#1787,.T.);
#2262=ORIENTED_EDGE('',*,*,#1792,.T.);
#2263=ORIENTED_EDGE('',*,*,#1688,.F.);
#2264=ORIENTED_EDGE('',*,*,#1793,.T.);
#2265=ORIENTED_EDGE('',*,*,#1790,.T.);
#2266=ORIENTED_EDGE('',*,*,#1794,.T.);
#2267=ORIENTED_EDGE('',*,*,#1752,.F.);
#2268=ORIENTED_EDGE('',*,*,#1795,.T.);
#2269=ORIENTED_EDGE('',*,*,#1766,.T.);
#2270=ORIENTED_EDGE('',*,*,#1796,.T.);
#2271=ORIENTED_EDGE('',*,*,#1695,.T.);
#2272=ORIENTED_EDGE('',*,*,#1797,.T.);
#2273=ORIENTED_EDGE('',*,*,#1663,.F.);
#2274=ORIENTED_EDGE('',*,*,#1798,.T.);
#2275=ORIENTED_EDGE('',*,*,#1762,.F.);
#2276=ORIENTED_EDGE('',*,*,#1799,.T.);
#2277=ORIENTED_EDGE('',*,*,#1755,.T.);
#2278=ORIENTED_EDGE('',*,*,#1728,.T.);
#2279=ORIENTED_EDGE('',*,*,#1725,.T.);
#2280=ORIENTED_EDGE('',*,*,#1722,.T.);
#2281=ORIENTED_EDGE('',*,*,#1697,.F.);
#2282=ORIENTED_EDGE('',*,*,#1800,.T.);
#2283=ORIENTED_EDGE('',*,*,#1689,.F.);
#2284=ORIENTED_EDGE('',*,*,#1794,.F.);
#2285=ORIENTED_EDGE('',*,*,#1792,.F.);
#2286=ORIENTED_EDGE('',*,*,#1789,.F.);
#2287=ORIENTED_EDGE('',*,*,#1687,.F.);
#2288=ORIENTED_EDGE('',*,*,#1801,.T.);
#2289=ORIENTED_EDGE('',*,*,#1699,.F.);
#2290=ORIENTED_EDGE('',*,*,#1721,.T.);
#2291=ORIENTED_EDGE('',*,*,#1724,.T.);
#2292=ORIENTED_EDGE('',*,*,#1727,.T.);
#2293=ORIENTED_EDGE('',*,*,#1754,.T.);
#2294=ORIENTED_EDGE('',*,*,#1802,.T.);
#2295=ORIENTED_EDGE('',*,*,#1764,.F.);
#2296=ORIENTED_EDGE('',*,*,#1788,.F.);
#2297=ORIENTED_EDGE('',*,*,#1791,.F.);
#2298=ORIENTED_EDGE('',*,*,#1793,.F.);
#2299=ORIENTED_EDGE('',*,*,#1733,.T.);
#2300=ORIENTED_EDGE('',*,*,#1803,.T.);
#2301=ORIENTED_EDGE('',*,*,#1785,.F.);
#2302=ORIENTED_EDGE('',*,*,#1804,.T.);
#2303=ORIENTED_EDGE('',*,*,#1769,.F.);
#2304=ORIENTED_EDGE('',*,*,#1805,.T.);
#2305=ORIENTED_EDGE('',*,*,#1749,.T.);
#2306=ORIENTED_EDGE('',*,*,#1806,.F.);
#2307=ORIENTED_EDGE('',*,*,#1806,.T.);
#2308=ORIENTED_EDGE('',*,*,#1748,.T.);
#2309=ORIENTED_EDGE('',*,*,#1807,.F.);
#2310=ORIENTED_EDGE('',*,*,#1770,.F.);
#2311=ORIENTED_EDGE('',*,*,#1747,.T.);
#2312=ORIENTED_EDGE('',*,*,#1808,.T.);
#2313=ORIENTED_EDGE('',*,*,#1771,.F.);
#2314=ORIENTED_EDGE('',*,*,#1807,.T.);
#2315=ORIENTED_EDGE('',*,*,#1773,.F.);
#2316=ORIENTED_EDGE('',*,*,#1809,.T.);
#2317=ORIENTED_EDGE('',*,*,#1745,.T.);
#2318=ORIENTED_EDGE('',*,*,#1810,.F.);
#2319=ORIENTED_EDGE('',*,*,#1810,.T.);
#2320=ORIENTED_EDGE('',*,*,#1744,.T.);
#2321=ORIENTED_EDGE('',*,*,#1811,.F.);
#2322=ORIENTED_EDGE('',*,*,#1774,.F.);
#2323=ORIENTED_EDGE('',*,*,#1743,.T.);
#2324=ORIENTED_EDGE('',*,*,#1812,.T.);
#2325=ORIENTED_EDGE('',*,*,#1775,.F.);
#2326=ORIENTED_EDGE('',*,*,#1811,.T.);
#2327=ORIENTED_EDGE('',*,*,#1741,.T.);
#2328=ORIENTED_EDGE('',*,*,#1813,.T.);
#2329=ORIENTED_EDGE('',*,*,#1777,.F.);
#2330=ORIENTED_EDGE('',*,*,#1814,.T.);
#2331=ORIENTED_EDGE('',*,*,#1779,.F.);
#2332=ORIENTED_EDGE('',*,*,#1815,.T.);
#2333=ORIENTED_EDGE('',*,*,#1739,.T.);
#2334=ORIENTED_EDGE('',*,*,#1816,.F.);
#2335=ORIENTED_EDGE('',*,*,#1816,.T.);
#2336=ORIENTED_EDGE('',*,*,#1738,.T.);
#2337=ORIENTED_EDGE('',*,*,#1817,.F.);
#2338=ORIENTED_EDGE('',*,*,#1780,.F.);
#2339=ORIENTED_EDGE('',*,*,#1737,.T.);
#2340=ORIENTED_EDGE('',*,*,#1818,.T.);
#2341=ORIENTED_EDGE('',*,*,#1781,.F.);
#2342=ORIENTED_EDGE('',*,*,#1817,.T.);
#2343=ORIENTED_EDGE('',*,*,#1783,.F.);
#2344=ORIENTED_EDGE('',*,*,#1819,.T.);
#2345=ORIENTED_EDGE('',*,*,#1735,.T.);
#2346=ORIENTED_EDGE('',*,*,#1820,.F.);
#2347=ORIENTED_EDGE('',*,*,#1820,.T.);
#2348=ORIENTED_EDGE('',*,*,#1734,.T.);
#2349=ORIENTED_EDGE('',*,*,#1804,.F.);
#2350=ORIENTED_EDGE('',*,*,#1784,.F.);
#2351=ORIENTED_EDGE('',*,*,#1821,.F.);
#2352=ORIENTED_EDGE('',*,*,#1718,.F.);
#2353=ORIENTED_EDGE('',*,*,#1822,.T.);
#2354=ORIENTED_EDGE('',*,*,#1668,.F.);
#2355=ORIENTED_EDGE('',*,*,#1717,.F.);
#2356=ORIENTED_EDGE('',*,*,#1823,.T.);
#2357=ORIENTED_EDGE('',*,*,#1669,.F.);
#2358=ORIENTED_EDGE('',*,*,#1822,.F.);
#2359=ORIENTED_EDGE('',*,*,#1671,.F.);
#2360=ORIENTED_EDGE('',*,*,#1824,.T.);
#2361=ORIENTED_EDGE('',*,*,#1715,.F.);
#2362=ORIENTED_EDGE('',*,*,#1825,.T.);
#2363=ORIENTED_EDGE('',*,*,#1825,.F.);
#2364=ORIENTED_EDGE('',*,*,#1714,.F.);
#2365=ORIENTED_EDGE('',*,*,#1826,.T.);
#2366=ORIENTED_EDGE('',*,*,#1672,.F.);
#2367=ORIENTED_EDGE('',*,*,#1713,.F.);
#2368=ORIENTED_EDGE('',*,*,#1827,.T.);
#2369=ORIENTED_EDGE('',*,*,#1673,.F.);
#2370=ORIENTED_EDGE('',*,*,#1826,.F.);
#2371=ORIENTED_EDGE('',*,*,#1675,.F.);
#2372=ORIENTED_EDGE('',*,*,#1828,.T.);
#2373=ORIENTED_EDGE('',*,*,#1711,.F.);
#2374=ORIENTED_EDGE('',*,*,#1829,.T.);
#2375=ORIENTED_EDGE('',*,*,#1677,.F.);
#2376=ORIENTED_EDGE('',*,*,#1830,.T.);
#2377=ORIENTED_EDGE('',*,*,#1709,.F.);
#2378=ORIENTED_EDGE('',*,*,#1831,.T.);
#2379=ORIENTED_EDGE('',*,*,#1831,.F.);
#2380=ORIENTED_EDGE('',*,*,#1708,.F.);
#2381=ORIENTED_EDGE('',*,*,#1832,.T.);
#2382=ORIENTED_EDGE('',*,*,#1678,.F.);
#2383=ORIENTED_EDGE('',*,*,#1707,.F.);
#2384=ORIENTED_EDGE('',*,*,#1833,.T.);
#2385=ORIENTED_EDGE('',*,*,#1679,.F.);
#2386=ORIENTED_EDGE('',*,*,#1832,.F.);
#2387=ORIENTED_EDGE('',*,*,#1681,.F.);
#2388=ORIENTED_EDGE('',*,*,#1834,.T.);
#2389=ORIENTED_EDGE('',*,*,#1705,.F.);
#2390=ORIENTED_EDGE('',*,*,#1835,.T.);
#2391=ORIENTED_EDGE('',*,*,#1835,.F.);
#2392=ORIENTED_EDGE('',*,*,#1704,.F.);
#2393=ORIENTED_EDGE('',*,*,#1836,.T.);
#2394=ORIENTED_EDGE('',*,*,#1682,.F.);
#2395=ORIENTED_EDGE('',*,*,#1703,.F.);
#2396=ORIENTED_EDGE('',*,*,#1837,.T.);
#2397=ORIENTED_EDGE('',*,*,#1683,.F.);
#2398=ORIENTED_EDGE('',*,*,#1836,.F.);
#2399=ORIENTED_EDGE('',*,*,#1667,.F.);
#2400=ORIENTED_EDGE('',*,*,#1838,.T.);
#2401=ORIENTED_EDGE('',*,*,#1719,.F.);
#2402=ORIENTED_EDGE('',*,*,#1821,.T.);
#2403=ORIENTED_EDGE('',*,*,#1776,.F.);
#2404=ORIENTED_EDGE('',*,*,#1812,.F.);
#2405=ORIENTED_EDGE('',*,*,#1742,.F.);
#2406=ORIENTED_EDGE('',*,*,#1814,.F.);
#2407=ORIENTED_EDGE('',*,*,#1778,.F.);
#2408=ORIENTED_EDGE('',*,*,#1813,.F.);
#2409=ORIENTED_EDGE('',*,*,#1740,.F.);
#2410=ORIENTED_EDGE('',*,*,#1815,.F.);
#2411=ORIENTED_EDGE('',*,*,#1782,.F.);
#2412=ORIENTED_EDGE('',*,*,#1818,.F.);
#2413=ORIENTED_EDGE('',*,*,#1736,.F.);
#2414=ORIENTED_EDGE('',*,*,#1819,.F.);
#2415=ORIENTED_EDGE('',*,*,#1772,.F.);
#2416=ORIENTED_EDGE('',*,*,#1808,.F.);
#2417=ORIENTED_EDGE('',*,*,#1746,.F.);
#2418=ORIENTED_EDGE('',*,*,#1809,.F.);
#2419=ORIENTED_EDGE('',*,*,#1710,.F.);
#2420=ORIENTED_EDGE('',*,*,#1830,.F.);
#2421=ORIENTED_EDGE('',*,*,#1676,.F.);
#2422=ORIENTED_EDGE('',*,*,#1829,.F.);
#2423=ORIENTED_EDGE('',*,*,#1706,.F.);
#2424=ORIENTED_EDGE('',*,*,#1834,.F.);
#2425=ORIENTED_EDGE('',*,*,#1680,.F.);
#2426=ORIENTED_EDGE('',*,*,#1833,.F.);
#2427=ORIENTED_EDGE('',*,*,#1716,.F.);
#2428=ORIENTED_EDGE('',*,*,#1824,.F.);
#2429=ORIENTED_EDGE('',*,*,#1670,.F.);
#2430=ORIENTED_EDGE('',*,*,#1823,.F.);
#2431=ORIENTED_EDGE('',*,*,#1712,.F.);
#2432=ORIENTED_EDGE('',*,*,#1828,.F.);
#2433=ORIENTED_EDGE('',*,*,#1674,.F.);
#2434=ORIENTED_EDGE('',*,*,#1827,.F.);
#2435=ORIENTED_EDGE('',*,*,#1768,.F.);
#2436=ORIENTED_EDGE('',*,*,#1654,.F.);
#2437=ORIENTED_EDGE('',*,*,#1750,.F.);
#2438=ORIENTED_EDGE('',*,*,#1805,.F.);
#2439=ORIENTED_EDGE('',*,*,#1786,.F.);
#2440=ORIENTED_EDGE('',*,*,#1803,.F.);
#2441=ORIENTED_EDGE('',*,*,#1732,.F.);
#2442=ORIENTED_EDGE('',*,*,#1759,.F.);
#2443=ORIENTED_EDGE('',*,*,#1720,.F.);
#2444=ORIENTED_EDGE('',*,*,#1838,.F.);
#2445=ORIENTED_EDGE('',*,*,#1666,.F.);
#2446=ORIENTED_EDGE('',*,*,#1693,.F.);
#2447=ORIENTED_EDGE('',*,*,#1702,.F.);
#2448=ORIENTED_EDGE('',*,*,#1650,.F.);
#2449=ORIENTED_EDGE('',*,*,#1684,.F.);
#2450=ORIENTED_EDGE('',*,*,#1837,.F.);
#2451=ORIENTED_EDGE('',*,*,#1760,.F.);
#2452=ORIENTED_EDGE('',*,*,#1757,.F.);
#2453=ORIENTED_EDGE('',*,*,#1730,.F.);
#2454=ORIENTED_EDGE('',*,*,#1656,.F.);
#2455=ORIENTED_EDGE('',*,*,#1761,.F.);
#2456=ORIENTED_EDGE('',*,*,#1658,.F.);
#2457=ORIENTED_EDGE('',*,*,#1756,.F.);
#2458=ORIENTED_EDGE('',*,*,#1799,.F.);
#2459=ORIENTED_EDGE('',*,*,#1694,.F.);
#2460=ORIENTED_EDGE('',*,*,#1691,.F.);
#2461=ORIENTED_EDGE('',*,*,#1664,.F.);
#2462=ORIENTED_EDGE('',*,*,#1797,.F.);
#2463=ORIENTED_EDGE('',*,*,#1690,.F.);
#2464=ORIENTED_EDGE('',*,*,#1800,.F.);
#2465=ORIENTED_EDGE('',*,*,#1696,.F.);
#2466=ORIENTED_EDGE('',*,*,#1798,.F.);
#2467=ORIENTED_EDGE('',*,*,#1701,.F.);
#2468=ORIENTED_EDGE('',*,*,#1660,.F.);
#2469=ORIENTED_EDGE('',*,*,#1685,.F.);
#2470=ORIENTED_EDGE('',*,*,#1648,.F.);
#2471=ORIENTED_EDGE('',*,*,#1686,.F.);
#2472=ORIENTED_EDGE('',*,*,#1662,.F.);
#2473=ORIENTED_EDGE('',*,*,#1700,.F.);
#2474=ORIENTED_EDGE('',*,*,#1801,.F.);
#2475=ORIENTED_EDGE('',*,*,#1767,.F.);
#2476=ORIENTED_EDGE('',*,*,#1795,.F.);
#2477=ORIENTED_EDGE('',*,*,#1751,.F.);
#2478=ORIENTED_EDGE('',*,*,#1652,.F.);
#2479=ORIENTED_EDGE('',*,*,#1753,.F.);
#2480=ORIENTED_EDGE('',*,*,#1796,.F.);
#2481=ORIENTED_EDGE('',*,*,#1765,.F.);
#2482=ORIENTED_EDGE('',*,*,#1802,.F.);
#3003=PLANE('',#3382);
#3004=PLANE('',#3383);
#3005=PLANE('',#3384);
#3006=PLANE('',#3385);
#3007=PLANE('',#3386);
#3008=PLANE('',#3391);
#3009=PLANE('',#3392);
#3010=PLANE('',#3400);
#3011=PLANE('',#3404);
#3012=PLANE('',#3409);
#3013=PLANE('',#3410);
#3014=PLANE('',#3418);
#3015=PLANE('',#3422);
#3016=PLANE('',#3423);
#3017=PLANE('',#3424);
#3018=PLANE('',#3425);
#3019=PLANE('',#3426);
#3020=PLANE('',#3427);
#3021=PLANE('',#3428);
#3022=PLANE('',#3429);
#3023=PLANE('',#3430);
#3024=PLANE('',#3431);
#3025=PLANE('',#3432);
#3026=PLANE('',#3433);
#3027=PLANE('',#3434);
#3028=PLANE('',#3435);
#3029=PLANE('',#3436);
#3030=PLANE('',#3437);
#3031=PLANE('',#3438);
#3032=PLANE('',#3439);
#3033=PLANE('',#3440);
#3034=PLANE('',#3441);
#3035=PLANE('',#3442);
#3036=PLANE('',#3443);
#3037=PLANE('',#3444);
#3038=PLANE('',#3445);
#3039=PLANE('',#3446);
#3040=PLANE('',#3447);
#3041=PLANE('',#3448);
#3042=PLANE('',#3449);
#3043=PLANE('',#3450);
#3044=PLANE('',#3451);
#3045=PLANE('',#3452);
#3046=PLANE('',#3453);
#3047=PLANE('',#3454);
#3048=PLANE('',#3455);
#3049=PLANE('',#3456);
#3050=PLANE('',#3457);
#3051=PLANE('',#3458);
#3052=PLANE('',#3459);
#3053=PLANE('',#3460);
#3054=PLANE('',#3461);
#3055=PLANE('',#3462);
#3056=PLANE('',#3463);
#3131=ADVANCED_FACE('',(#281),#3003,.T.);
#3132=ADVANCED_FACE('',(#282),#3004,.T.);
#3133=ADVANCED_FACE('',(#283),#3005,.T.);
#3134=ADVANCED_FACE('',(#284),#3006,.T.);
#3135=ADVANCED_FACE('',(#285),#3007,.F.);
#3136=ADVANCED_FACE('',(#286),#3008,.T.);
#3137=ADVANCED_FACE('',(#287),#3009,.T.);
#3138=ADVANCED_FACE('',(#288),#145,.T.);
#3139=ADVANCED_FACE('',(#289),#3010,.T.);
#3140=ADVANCED_FACE('',(#290),#146,.T.);
#3141=ADVANCED_FACE('',(#291),#3011,.T.);
#3142=ADVANCED_FACE('',(#292),#3012,.T.);
#3143=ADVANCED_FACE('',(#293),#3013,.F.);
#3144=ADVANCED_FACE('',(#294),#147,.F.);
#3145=ADVANCED_FACE('',(#295),#3014,.F.);
#3146=ADVANCED_FACE('',(#296),#148,.F.);
#3147=ADVANCED_FACE('',(#297),#3015,.T.);
#3148=ADVANCED_FACE('',(#298),#3016,.F.);
#3149=ADVANCED_FACE('',(#299),#3017,.F.);
#3150=ADVANCED_FACE('',(#300),#3018,.F.);
#3151=ADVANCED_FACE('',(#301),#3019,.F.);
#3152=ADVANCED_FACE('',(#302),#3020,.F.);
#3153=ADVANCED_FACE('',(#303),#3021,.F.);
#3154=ADVANCED_FACE('',(#304),#3022,.F.);
#3155=ADVANCED_FACE('',(#305),#3023,.F.);
#3156=ADVANCED_FACE('',(#306),#3024,.F.);
#3157=ADVANCED_FACE('',(#307),#3025,.F.);
#3158=ADVANCED_FACE('',(#308),#3026,.F.);
#3159=ADVANCED_FACE('',(#309),#3027,.F.);
#3160=ADVANCED_FACE('',(#310),#3028,.F.);
#3161=ADVANCED_FACE('',(#311),#3029,.F.);
#3162=ADVANCED_FACE('',(#312),#3030,.F.);
#3163=ADVANCED_FACE('',(#313),#3031,.F.);
#3164=ADVANCED_FACE('',(#314),#3032,.F.);
#3165=ADVANCED_FACE('',(#315),#3033,.F.);
#3166=ADVANCED_FACE('',(#316),#3034,.F.);
#3167=ADVANCED_FACE('',(#317),#3035,.F.);
#3168=ADVANCED_FACE('',(#318),#3036,.F.);
#3169=ADVANCED_FACE('',(#319),#3037,.F.);
#3170=ADVANCED_FACE('',(#320),#3038,.F.);
#3171=ADVANCED_FACE('',(#321),#3039,.F.);
#3172=ADVANCED_FACE('',(#322),#3040,.F.);
#3173=ADVANCED_FACE('',(#323),#3041,.F.);
#3174=ADVANCED_FACE('',(#324),#3042,.F.);
#3175=ADVANCED_FACE('',(#325),#3043,.F.);
#3176=ADVANCED_FACE('',(#326),#3044,.F.);
#3177=ADVANCED_FACE('',(#327),#3045,.F.);
#3178=ADVANCED_FACE('',(#328),#3046,.F.);
#3179=ADVANCED_FACE('',(#329),#3047,.F.);
#3180=ADVANCED_FACE('',(#330),#3048,.F.);
#3181=ADVANCED_FACE('',(#331),#3049,.F.);
#3182=ADVANCED_FACE('',(#332),#3050,.F.);
#3183=ADVANCED_FACE('',(#333),#3051,.F.);
#3184=ADVANCED_FACE('',(#334),#3052,.F.);
#3185=ADVANCED_FACE('',(#335),#3053,.T.);
#3186=ADVANCED_FACE('',(#336),#3054,.T.);
#3187=ADVANCED_FACE('',(#337),#3055,.T.);
#3188=ADVANCED_FACE('',(#338),#3056,.T.);
#3189=ADVANCED_FACE('',(#339),#149,.T.);
#3190=ADVANCED_FACE('',(#340),#150,.T.);
#3191=ADVANCED_FACE('',(#341),#151,.T.);
#3192=ADVANCED_FACE('',(#342),#152,.T.);
#3193=ADVANCED_FACE('',(#343),#153,.T.);
#3194=ADVANCED_FACE('',(#344),#154,.T.);
#3195=ADVANCED_FACE('',(#345),#155,.T.);
#3196=ADVANCED_FACE('',(#346),#156,.T.);
#3307=CLOSED_SHELL('',(#3131,#3132,#3133,#3134,#3135,#3136,#3137,#3138,
#3139,#3140,#3141,#3142,#3143,#3144,#3145,#3146,#3147,#3148,#3149,#3150,
#3151,#3152,#3153,#3154,#3155,#3156,#3157,#3158,#3159,#3160,#3161,#3162,
#3163,#3164,#3165,#3166,#3167,#3168,#3169,#3170,#3171,#3172,#3173,#3174,
#3175,#3176,#3177,#3178,#3179,#3180,#3181,#3182,#3183,#3184,#3185,#3186,
#3187,#3188,#3189,#3190,#3191,#3192,#3193,#3194,#3195,#3196));
#3381=AXIS2_PLACEMENT_3D('',#4640,#3683,#3684);
#3382=AXIS2_PLACEMENT_3D('',#4641,#3685,#3686);
#3383=AXIS2_PLACEMENT_3D('',#4650,#3691,#3692);
#3384=AXIS2_PLACEMENT_3D('',#4659,#3697,#3698);
#3385=AXIS2_PLACEMENT_3D('',#4668,#3703,#3704);
#3386=AXIS2_PLACEMENT_3D('',#4677,#3709,#3710);
#3387=AXIS2_PLACEMENT_3D('',#4682,#3712,#3713);
#3388=AXIS2_PLACEMENT_3D('',#4722,#3734,#3735);
#3389=AXIS2_PLACEMENT_3D('',#4724,#3736,#3737);
#3390=AXIS2_PLACEMENT_3D('',#4731,#3741,#3742);
#3391=AXIS2_PLACEMENT_3D('',#4732,#3743,#3744);
#3392=AXIS2_PLACEMENT_3D('',#4738,#3748,#3749);
#3393=AXIS2_PLACEMENT_3D('',#4740,#3750,#3751);
#3394=AXIS2_PLACEMENT_3D('',#4744,#3753,#3754);
#3395=AXIS2_PLACEMENT_3D('',#4751,#3758,#3759);
#3396=AXIS2_PLACEMENT_3D('',#4752,#3760,#3761);
#3397=AXIS2_PLACEMENT_3D('',#4790,#3781,#3782);
#3398=AXIS2_PLACEMENT_3D('',#4792,#3783,#3784);
#3399=AXIS2_PLACEMENT_3D('',#4794,#3785,#3786);
#3400=AXIS2_PLACEMENT_3D('',#4796,#3788,#3789);
#3401=AXIS2_PLACEMENT_3D('',#4802,#3793,#3794);
#3402=AXIS2_PLACEMENT_3D('',#4804,#3795,#3796);
#3403=AXIS2_PLACEMENT_3D('',#4806,#3797,#3798);
#3404=AXIS2_PLACEMENT_3D('',#4808,#3800,#3801);
#3405=AXIS2_PLACEMENT_3D('',#4810,#3802,#3803);
#3406=AXIS2_PLACEMENT_3D('',#4851,#3824,#3825);
#3407=AXIS2_PLACEMENT_3D('',#4855,#3827,#3828);
#3408=AXIS2_PLACEMENT_3D('',#4859,#3831,#3832);
#3409=AXIS2_PLACEMENT_3D('',#4860,#3833,#3834);
#3410=AXIS2_PLACEMENT_3D('',#4866,#3838,#3839);
#3411=AXIS2_PLACEMENT_3D('',#4867,#3840,#3841);
#3412=AXIS2_PLACEMENT_3D('',#4869,#3842,#3843);
#3413=AXIS2_PLACEMENT_3D('',#4877,#3847,#3848);
#3414=AXIS2_PLACEMENT_3D('',#4880,#3850,#3851);
#3415=AXIS2_PLACEMENT_3D('',#4918,#3871,#3872);
#3416=AXIS2_PLACEMENT_3D('',#4922,#3874,#3875);
#3417=AXIS2_PLACEMENT_3D('',#4923,#3876,#3877);
#3418=AXIS2_PLACEMENT_3D('',#4924,#3878,#3879);
#3419=AXIS2_PLACEMENT_3D('',#4930,#3883,#3884);
#3420=AXIS2_PLACEMENT_3D('',#4931,#3885,#3886);
#3421=AXIS2_PLACEMENT_3D('',#4932,#3887,#3888);
#3422=AXIS2_PLACEMENT_3D('',#4933,#3889,#3890);
#3423=AXIS2_PLACEMENT_3D('',#4936,#3893,#3894);
#3424=AXIS2_PLACEMENT_3D('',#4939,#3897,#3898);
#3425=AXIS2_PLACEMENT_3D('',#4942,#3901,#3902);
#3426=AXIS2_PLACEMENT_3D('',#4945,#3905,#3906);
#3427=AXIS2_PLACEMENT_3D('',#4948,#3909,#3910);
#3428=AXIS2_PLACEMENT_3D('',#4951,#3913,#3914);
#3429=AXIS2_PLACEMENT_3D('',#4953,#3916,#3917);
#3430=AXIS2_PLACEMENT_3D('',#4955,#3919,#3920);
#3431=AXIS2_PLACEMENT_3D('',#4958,#3923,#3924);
#3432=AXIS2_PLACEMENT_3D('',#4960,#3926,#3927);
#3433=AXIS2_PLACEMENT_3D('',#4962,#3929,#3930);
#3434=AXIS2_PLACEMENT_3D('',#4965,#3933,#3934);
#3435=AXIS2_PLACEMENT_3D('',#4968,#3937,#3938);
#3436=AXIS2_PLACEMENT_3D('',#4970,#3940,#3941);
#3437=AXIS2_PLACEMENT_3D('',#4972,#3943,#3944);
#3438=AXIS2_PLACEMENT_3D('',#4975,#3947,#3948);
#3439=AXIS2_PLACEMENT_3D('',#4976,#3949,#3950);
#3440=AXIS2_PLACEMENT_3D('',#4979,#3953,#3954);
#3441=AXIS2_PLACEMENT_3D('',#4981,#3956,#3957);
#3442=AXIS2_PLACEMENT_3D('',#4984,#3960,#3961);
#3443=AXIS2_PLACEMENT_3D('',#4986,#3963,#3964);
#3444=AXIS2_PLACEMENT_3D('',#4988,#3966,#3967);
#3445=AXIS2_PLACEMENT_3D('',#4991,#3970,#3971);
#3446=AXIS2_PLACEMENT_3D('',#4994,#3974,#3975);
#3447=AXIS2_PLACEMENT_3D('',#4996,#3977,#3978);
#3448=AXIS2_PLACEMENT_3D('',#4998,#3980,#3981);
#3449=AXIS2_PLACEMENT_3D('',#5001,#3984,#3985);
#3450=AXIS2_PLACEMENT_3D('',#5003,#3987,#3988);
#3451=AXIS2_PLACEMENT_3D('',#5005,#3990,#3991);
#3452=AXIS2_PLACEMENT_3D('',#5007,#3993,#3994);
#3453=AXIS2_PLACEMENT_3D('',#5008,#3995,#3996);
#3454=AXIS2_PLACEMENT_3D('',#5009,#3997,#3998);
#3455=AXIS2_PLACEMENT_3D('',#5010,#3999,#4000);
#3456=AXIS2_PLACEMENT_3D('',#5011,#4001,#4002);
#3457=AXIS2_PLACEMENT_3D('',#5012,#4003,#4004);
#3458=AXIS2_PLACEMENT_3D('',#5013,#4005,#4006);
#3459=AXIS2_PLACEMENT_3D('',#5014,#4007,#4008);
#3460=AXIS2_PLACEMENT_3D('',#5015,#4009,#4010);
#3461=AXIS2_PLACEMENT_3D('',#5016,#4011,#4012);
#3462=AXIS2_PLACEMENT_3D('',#5017,#4013,#4014);
#3463=AXIS2_PLACEMENT_3D('',#5018,#4015,#4016);
#3464=AXIS2_PLACEMENT_3D('',#5019,#4017,#4018);
#3465=AXIS2_PLACEMENT_3D('',#5020,#4019,#4020);
#3466=AXIS2_PLACEMENT_3D('',#5021,#4021,#4022);
#3467=AXIS2_PLACEMENT_3D('',#5022,#4023,#4024);
#3468=AXIS2_PLACEMENT_3D('',#5023,#4025,#4026);
#3469=AXIS2_PLACEMENT_3D('',#5024,#4027,#4028);
#3470=AXIS2_PLACEMENT_3D('',#5025,#4029,#4030);
#3471=AXIS2_PLACEMENT_3D('',#5026,#4031,#4032);
#3683=DIRECTION('axis',(0.,0.,1.));
#3684=DIRECTION('refdir',(1.,0.,0.));
#3685=DIRECTION('center_axis',(-9.01019857023267E-31,-1.,0.));
#3686=DIRECTION('ref_axis',(1.,-9.01019857023267E-31,0.));
#3687=DIRECTION('',(0.,0.,-1.));
#3688=DIRECTION('',(-1.,9.01019857023267E-31,0.));
#3689=DIRECTION('',(0.,0.,-1.));
#3690=DIRECTION('',(1.,-9.01019857023267E-31,0.));
#3691=DIRECTION('center_axis',(0.,-1.,0.));
#3692=DIRECTION('ref_axis',(0.,0.,-1.));
#3693=DIRECTION('',(0.,0.,-1.));
#3694=DIRECTION('',(-1.,0.,0.));
#3695=DIRECTION('',(0.,0.,-1.));
#3696=DIRECTION('',(1.,0.,0.));
#3697=DIRECTION('center_axis',(0.,0.,-1.));
#3698=DIRECTION('ref_axis',(-1.,0.,0.));
#3699=DIRECTION('',(0.,1.,0.));
#3700=DIRECTION('',(-1.,0.,0.));
#3701=DIRECTION('',(0.,1.,0.));
#3702=DIRECTION('',(1.,0.,0.));
#3703=DIRECTION('center_axis',(0.,0.,1.));
#3704=DIRECTION('ref_axis',(1.,0.,0.));
#3705=DIRECTION('',(-3.46944695195361E-16,-1.,0.));
#3706=DIRECTION('',(1.,-9.01019857023267E-31,0.));
#3707=DIRECTION('',(-3.46944695195361E-16,-1.,0.));
#3708=DIRECTION('',(-1.,0.,0.));
#3709=DIRECTION('center_axis',(1.,-3.46944695195361E-16,0.));
#3710=DIRECTION('ref_axis',(3.46944695195361E-16,1.,0.));
#3711=DIRECTION('',(-3.46944695195361E-16,-1.,0.));
#3712=DIRECTION('center_axis',(-1.,3.46944695195361E-16,0.));
#3713=DIRECTION('ref_axis',(3.46944695195361E-16,1.,0.));
#3714=DIRECTION('',(0.,0.,-1.));
#3715=DIRECTION('',(2.4532694666934E-16,0.707106781186549,0.707106781186546));
#3716=DIRECTION('',(3.46944695195361E-16,1.,4.3841477367998E-16));
#3717=DIRECTION('',(2.27580604085849E-16,0.655956431204979,0.754798754874985));
#3718=DIRECTION('',(0.,0.,1.));
#3719=DIRECTION('',(2.4532694666934E-16,0.707106781186547,0.707106781186547));
#3720=DIRECTION('',(3.46944695195361E-16,1.,0.));
#3721=DIRECTION('',(0.,0.,1.));
#3722=DIRECTION('',(-3.46944695195361E-16,-1.,0.));
#3723=DIRECTION('',(-2.4532694666934E-16,-0.707106781186548,0.707106781186547));
#3724=DIRECTION('',(0.,0.,1.));
#3725=DIRECTION('',(2.4532694666934E-16,0.707106781186547,0.707106781186547));
#3726=DIRECTION('',(3.46944695195361E-16,1.,0.));
#3727=DIRECTION('',(0.,0.,1.));
#3728=DIRECTION('',(-3.46944695195361E-16,-1.,0.));
#3729=DIRECTION('',(-2.4532694666934E-16,-0.707106781186548,0.707106781186547));
#3730=DIRECTION('',(0.,-8.15936190770267E-17,1.));
#3731=DIRECTION('',(-1.82277714383761E-16,-0.525379741809059,0.85086786688454));
#3732=DIRECTION('',(-3.46944695195361E-16,-1.,0.));
#3733=DIRECTION('',(-2.4532694666934E-16,-0.707106781186548,0.707106781186547));
#3734=DIRECTION('center_axis',(-1.,3.46944695195361E-16,0.));
#3735=DIRECTION('ref_axis',(3.46944695195361E-16,1.,0.));
#3736=DIRECTION('center_axis',(-1.,3.46944695195361E-16,0.));
#3737=DIRECTION('ref_axis',(3.46944695195361E-16,1.,0.));
#3738=DIRECTION('',(2.05674862010263E-16,0.592817428421694,-0.805336883893622));
#3739=DIRECTION('',(0.,0.,-1.));
#3740=DIRECTION('',(-2.05674862010263E-16,-0.592817428421694,-0.805336883893622));
#3741=DIRECTION('center_axis',(-1.,3.46944695195361E-16,0.));
#3742=DIRECTION('ref_axis',(3.46944695195361E-16,1.,8.67361737988404E-16));
#3743=DIRECTION('center_axis',(-9.01019857023267E-31,-1.,0.));
#3744=DIRECTION('ref_axis',(1.,-9.01019857023267E-31,0.));
#3745=DIRECTION('',(1.,-9.01019857023267E-31,0.));
#3746=DIRECTION('',(0.,0.,-1.));
#3747=DIRECTION('',(-1.,9.01019857023267E-31,0.));
#3748=DIRECTION('center_axis',(1.,-3.46944695195361E-16,0.));
#3749=DIRECTION('ref_axis',(3.46944695195361E-16,1.,0.));
#3750=DIRECTION('center_axis',(1.,-3.46944695195361E-16,0.));
#3751=DIRECTION('ref_axis',(3.46944695195361E-16,1.,0.));
#3752=DIRECTION('',(-3.46944695195361E-16,-1.,0.));
#3753=DIRECTION('center_axis',(1.,-3.46944695195361E-16,0.));
#3754=DIRECTION('ref_axis',(3.46944695195361E-16,1.,0.));
#3755=DIRECTION('',(0.,0.592817428421694,0.805336883893622));
#3756=DIRECTION('',(0.,0.,-1.));
#3757=DIRECTION('',(0.,-0.592817428421694,0.805336883893622));
#3758=DIRECTION('center_axis',(1.,-3.46944695195361E-16,0.));
#3759=DIRECTION('ref_axis',(3.46944695195361E-16,1.,0.));
#3760=DIRECTION('center_axis',(1.,-3.46944695195361E-16,0.));
#3761=DIRECTION('ref_axis',(3.46944695195361E-16,1.,0.));
#3762=DIRECTION('',(2.4532694666934E-16,0.707106781186548,-0.707106781186547));
#3763=DIRECTION('',(0.,1.,0.));
#3764=DIRECTION('',(0.,0.525379741809059,-0.85086786688454));
#3765=DIRECTION('',(0.,8.15936190770267E-17,-1.));
#3766=DIRECTION('',(2.4532694666934E-16,0.707106781186548,-0.707106781186547));
#3767=DIRECTION('',(0.,1.,0.));
#3768=DIRECTION('',(0.,0.,-1.));
#3769=DIRECTION('',(0.,-1.,0.));
#3770=DIRECTION('',(-2.4532694666934E-16,-0.707106781186547,-0.707106781186547));
#3771=DIRECTION('',(0.,0.,-1.));
#3772=DIRECTION('',(2.4532694666934E-16,0.707106781186548,-0.707106781186547));
#3773=DIRECTION('',(0.,1.,0.));
#3774=DIRECTION('',(0.,0.,-1.));
#3775=DIRECTION('',(0.,-1.,0.));
#3776=DIRECTION('',(-2.4532694666934E-16,-0.707106781186547,-0.707106781186547));
#3777=DIRECTION('',(0.,0.,-1.));
#3778=DIRECTION('',(0.,-0.655956431204979,-0.754798754874985));
#3779=DIRECTION('',(0.,-1.,-4.3841477367998E-16));
#3780=DIRECTION('',(-2.4532694666934E-16,-0.707106781186549,-0.707106781186546));
#3781=DIRECTION('center_axis',(0.,0.,-1.));
#3782=DIRECTION('ref_axis',(-1.,0.,0.));
#3783=DIRECTION('center_axis',(-2.37922000563897E-14,0.805336883893611,
0.59281742842171));
#3784=DIRECTION('ref_axis',(4.37979299315037E-14,-0.59281742842171,0.805336883893611));
#3785=DIRECTION('center_axis',(3.26041260031985E-15,0.805336883893623,-0.592817428421693));
#3786=DIRECTION('ref_axis',(7.54167563526444E-14,0.592817428421693,0.805336883893623));
#3787=DIRECTION('',(0.,0.,-1.));
#3788=DIRECTION('center_axis',(0.,1.,0.));
#3789=DIRECTION('ref_axis',(0.,0.,1.));
#3790=DIRECTION('',(-1.,0.,0.));
#3791=DIRECTION('',(1.,0.,0.));
#3792=DIRECTION('',(0.,0.,-1.));
#3793=DIRECTION('center_axis',(0.,0.,-1.));
#3794=DIRECTION('ref_axis',(-1.,0.,0.));
#3795=DIRECTION('center_axis',(-1.44515585527699E-14,0.805336883893626,
0.59281742842169));
#3796=DIRECTION('ref_axis',(8.24431622240136E-14,-0.59281742842169,0.805336883893626));
#3797=DIRECTION('center_axis',(-4.05348593553306E-15,0.805336883893625,
-0.592817428421691));
#3798=DIRECTION('ref_axis',(2.27187123174103E-14,0.59281742842169,0.805336883893625));
#3799=DIRECTION('',(0.,0.,-1.));
#3800=DIRECTION('center_axis',(-1.,0.,0.));
#3801=DIRECTION('ref_axis',(0.,0.,1.));
#3802=DIRECTION('center_axis',(-1.,0.,0.));
#3803=DIRECTION('ref_axis',(0.,0.,1.));
#3804=DIRECTION('',(0.,0.,-1.));
#3805=DIRECTION('',(0.,0.707106781186549,0.707106781186546));
#3806=DIRECTION('',(0.,-1.,-4.3841477367998E-16));
#3807=DIRECTION('',(0.,-0.655956431204979,-0.754798754874985));
#3808=DIRECTION('',(0.,0.,-1.));
#3809=DIRECTION('',(0.,0.707106781186547,0.707106781186547));
#3810=DIRECTION('',(0.,-1.,0.));
#3811=DIRECTION('',(0.,0.,-1.));
#3812=DIRECTION('',(0.,1.,0.));
#3813=DIRECTION('',(0.,-0.707106781186548,0.707106781186547));
#3814=DIRECTION('',(0.,0.,-1.));
#3815=DIRECTION('',(0.,0.707106781186547,0.707106781186547));
#3816=DIRECTION('',(0.,-1.,0.));
#3817=DIRECTION('',(0.,0.,-1.));
#3818=DIRECTION('',(0.,1.,0.));
#3819=DIRECTION('',(0.,-0.707106781186548,0.707106781186547));
#3820=DIRECTION('',(0.,8.15936190770267E-17,-1.));
#3821=DIRECTION('',(0.,0.525379741809059,-0.85086786688454));
#3822=DIRECTION('',(0.,1.,0.));
#3823=DIRECTION('',(0.,-0.707106781186548,0.707106781186547));
#3824=DIRECTION('center_axis',(-1.,0.,0.));
#3825=DIRECTION('ref_axis',(0.,0.,1.));
#3826=DIRECTION('',(0.,1.,0.));
#3827=DIRECTION('center_axis',(-1.,0.,0.));
#3828=DIRECTION('ref_axis',(0.,0.,1.));
#3829=DIRECTION('',(0.,-0.592817428421694,0.805336883893622));
#3830=DIRECTION('',(0.,0.592817428421694,0.805336883893622));
#3831=DIRECTION('center_axis',(-1.,0.,0.));
#3832=DIRECTION('ref_axis',(0.,0.,1.));
#3833=DIRECTION('center_axis',(0.,-1.,0.));
#3834=DIRECTION('ref_axis',(0.,0.,-1.));
#3835=DIRECTION('',(1.,0.,0.));
#3836=DIRECTION('',(0.,0.,-1.));
#3837=DIRECTION('',(-1.,0.,0.));
#3838=DIRECTION('center_axis',(-1.,0.,0.));
#3839=DIRECTION('ref_axis',(0.,0.,1.));
#3840=DIRECTION('center_axis',(1.,0.,0.));
#3841=DIRECTION('ref_axis',(0.,0.,1.));
#3842=DIRECTION('center_axis',(1.,0.,0.));
#3843=DIRECTION('ref_axis',(0.,0.,1.));
#3844=DIRECTION('',(0.,0.592817428421694,0.805336883893622));
#3845=DIRECTION('',(0.,0.,-1.));
#3846=DIRECTION('',(0.,-0.592817428421694,0.805336883893622));
#3847=DIRECTION('center_axis',(1.,0.,0.));
#3848=DIRECTION('ref_axis',(0.,1.80411241501588E-14,1.));
#3849=DIRECTION('',(0.,1.,0.));
#3850=DIRECTION('center_axis',(1.,0.,0.));
#3851=DIRECTION('ref_axis',(0.,0.,1.));
#3852=DIRECTION('',(0.,0.707106781186548,-0.707106781186547));
#3853=DIRECTION('',(0.,1.,0.));
#3854=DIRECTION('',(0.,0.525379741809059,-0.85086786688454));
#3855=DIRECTION('',(0.,8.15936190770267E-17,-1.));
#3856=DIRECTION('',(0.,0.707106781186548,-0.707106781186547));
#3857=DIRECTION('',(0.,1.,0.));
#3858=DIRECTION('',(0.,0.,-1.));
#3859=DIRECTION('',(0.,-1.,0.));
#3860=DIRECTION('',(0.,-0.707106781186547,-0.707106781186547));
#3861=DIRECTION('',(0.,0.,-1.));
#3862=DIRECTION('',(0.,0.707106781186548,-0.707106781186547));
#3863=DIRECTION('',(0.,1.,0.));
#3864=DIRECTION('',(0.,0.,-1.));
#3865=DIRECTION('',(0.,-1.,0.));
#3866=DIRECTION('',(0.,-0.707106781186547,-0.707106781186547));
#3867=DIRECTION('',(0.,0.,-1.));
#3868=DIRECTION('',(0.,-0.655956431204979,-0.754798754874985));
#3869=DIRECTION('',(0.,-1.,-4.3841477367998E-16));
#3870=DIRECTION('',(0.,-0.707106781186549,-0.707106781186546));
#3871=DIRECTION('center_axis',(0.,0.,-1.));
#3872=DIRECTION('ref_axis',(-1.,0.,0.));
#3873=DIRECTION('',(0.,0.,-1.));
#3874=DIRECTION('center_axis',(-6.87444778888498E-14,0.805336883893647,
0.592817428421661));
#3875=DIRECTION('ref_axis',(4.06950357233023E-13,-0.592817428421661,0.805336883893647));
#3876=DIRECTION('center_axis',(2.2006022666971E-14,0.805336883893619,-0.592817428421699));
#3877=DIRECTION('ref_axis',(1.87317276168279E-13,0.592817428421699,0.805336883893618));
#3878=DIRECTION('center_axis',(0.,1.,0.));
#3879=DIRECTION('ref_axis',(0.,0.,1.));
#3880=DIRECTION('',(0.,0.,-1.));
#3881=DIRECTION('',(-1.,0.,0.));
#3882=DIRECTION('',(1.,0.,0.));
#3883=DIRECTION('center_axis',(0.,0.,-1.));
#3884=DIRECTION('ref_axis',(-1.,0.,0.));
#3885=DIRECTION('center_axis',(-5.02438393635322E-14,0.805336883893605,
0.592817428421718));
#3886=DIRECTION('ref_axis',(1.40144780436978E-12,-0.592817428421718,0.805336883893605));
#3887=DIRECTION('center_axis',(-8.56871679067861E-15,0.805336883893636,
-0.592817428421675));
#3888=DIRECTION('ref_axis',(1.35125821358047E-13,0.592817428421675,0.805336883893636));
#3889=DIRECTION('center_axis',(0.,0.,1.));
#3890=DIRECTION('ref_axis',(1.,0.,0.));
#3891=DIRECTION('',(1.,0.,0.));
#3892=DIRECTION('',(-1.,0.,0.));
#3893=DIRECTION('center_axis',(0.,0.,1.));
#3894=DIRECTION('ref_axis',(1.,0.,0.));
#3895=DIRECTION('',(-1.,9.01019857023267E-31,0.));
#3896=DIRECTION('',(1.,0.,0.));
#3897=DIRECTION('center_axis',(0.,-0.805336883893622,0.592817428421694));
#3898=DIRECTION('ref_axis',(0.,-0.592817428421694,-0.805336883893622));
#3899=DIRECTION('',(-1.,0.,0.));
#3900=DIRECTION('',(-1.,0.,0.));
#3901=DIRECTION('center_axis',(0.,-0.805336883893622,-0.592817428421694));
#3902=DIRECTION('ref_axis',(0.,0.592817428421694,-0.805336883893622));
#3903=DIRECTION('',(1.,0.,0.));
#3904=DIRECTION('',(1.,0.,0.));
#3905=DIRECTION('center_axis',(0.,4.3841477367998E-16,-1.));
#3906=DIRECTION('ref_axis',(0.,1.,4.3841477367998E-16));
#3907=DIRECTION('',(1.,0.,0.));
#3908=DIRECTION('',(-1.,0.,0.));
#3909=DIRECTION('center_axis',(0.,0.,1.));
#3910=DIRECTION('ref_axis',(1.,0.,0.));
#3911=DIRECTION('',(-1.,0.,0.));
#3912=DIRECTION('',(-1.,0.,0.));
#3913=DIRECTION('center_axis',(0.,0.85086786688454,0.525379741809059));
#3914=DIRECTION('ref_axis',(0.,-0.525379741809059,0.85086786688454));
#3915=DIRECTION('',(-1.,0.,0.));
#3916=DIRECTION('center_axis',(0.,1.,8.15936190770267E-17));
#3917=DIRECTION('ref_axis',(0.,-8.15936190770267E-17,1.));
#3918=DIRECTION('',(1.,0.,0.));
#3919=DIRECTION('center_axis',(0.,0.,1.));
#3920=DIRECTION('ref_axis',(1.,0.,0.));
#3921=DIRECTION('',(-1.,0.,0.));
#3922=DIRECTION('',(-1.,0.,0.));
#3923=DIRECTION('center_axis',(0.,1.,0.));
#3924=DIRECTION('ref_axis',(0.,0.,1.));
#3925=DIRECTION('',(-1.,0.,0.));
#3926=DIRECTION('center_axis',(0.,0.,-1.));
#3927=DIRECTION('ref_axis',(-1.,0.,0.));
#3928=DIRECTION('',(1.,0.,0.));
#3929=DIRECTION('center_axis',(0.,1.,0.));
#3930=DIRECTION('ref_axis',(0.,0.,1.));
#3931=DIRECTION('',(1.,0.,0.));
#3932=DIRECTION('',(-1.,0.,0.));
#3933=DIRECTION('center_axis',(0.,0.,1.));
#3934=DIRECTION('ref_axis',(1.,0.,0.));
#3935=DIRECTION('',(-1.,0.,0.));
#3936=DIRECTION('',(-1.,0.,0.));
#3937=DIRECTION('center_axis',(0.,1.,0.));
#3938=DIRECTION('ref_axis',(0.,0.,1.));
#3939=DIRECTION('',(-1.,0.,0.));
#3940=DIRECTION('center_axis',(0.,0.,-1.));
#3941=DIRECTION('ref_axis',(-1.,0.,0.));
#3942=DIRECTION('',(1.,0.,0.));
#3943=DIRECTION('center_axis',(0.,1.,0.));
#3944=DIRECTION('ref_axis',(0.,0.,1.));
#3945=DIRECTION('',(-1.,0.,0.));
#3946=DIRECTION('',(-1.,0.,0.));
#3947=DIRECTION('center_axis',(0.,0.754798754874985,-0.655956431204979));
#3948=DIRECTION('ref_axis',(0.,0.655956431204979,0.754798754874985));
#3949=DIRECTION('center_axis',(0.,0.754798754874985,-0.655956431204979));
#3950=DIRECTION('ref_axis',(0.,0.655956431204979,0.754798754874985));
#3951=DIRECTION('',(-1.,0.,0.));
#3952=DIRECTION('',(-1.,0.,0.));
#3953=DIRECTION('center_axis',(0.,1.,0.));
#3954=DIRECTION('ref_axis',(0.,0.,1.));
#3955=DIRECTION('',(-1.,0.,0.));
#3956=DIRECTION('center_axis',(0.,0.,-1.));
#3957=DIRECTION('ref_axis',(-1.,0.,0.));
#3958=DIRECTION('',(1.,0.,0.));
#3959=DIRECTION('',(-1.,0.,0.));
#3960=DIRECTION('center_axis',(0.,1.,0.));
#3961=DIRECTION('ref_axis',(0.,0.,1.));
#3962=DIRECTION('',(-1.,0.,0.));
#3963=DIRECTION('center_axis',(0.,0.,1.));
#3964=DIRECTION('ref_axis',(1.,0.,0.));
#3965=DIRECTION('',(-1.,0.,0.));
#3966=DIRECTION('center_axis',(0.,1.,0.));
#3967=DIRECTION('ref_axis',(0.,0.,1.));
#3968=DIRECTION('',(1.,0.,0.));
#3969=DIRECTION('',(-1.,0.,0.));
#3970=DIRECTION('center_axis',(0.,0.,-1.));
#3971=DIRECTION('ref_axis',(-1.,0.,0.));
#3972=DIRECTION('',(1.,0.,0.));
#3973=DIRECTION('',(-1.,0.,0.));
#3974=DIRECTION('center_axis',(0.,1.,0.));
#3975=DIRECTION('ref_axis',(0.,0.,1.));
#3976=DIRECTION('',(-1.,0.,0.));
#3977=DIRECTION('center_axis',(0.,0.,1.));
#3978=DIRECTION('ref_axis',(1.,0.,0.));
#3979=DIRECTION('',(-1.,0.,0.));
#3980=DIRECTION('center_axis',(0.,1.,8.15936190770267E-17));
#3981=DIRECTION('ref_axis',(0.,-8.15936190770267E-17,1.));
#3982=DIRECTION('',(1.,0.,0.));
#3983=DIRECTION('',(-1.,0.,0.));
#3984=DIRECTION('center_axis',(0.,0.85086786688454,0.525379741809059));
#3985=DIRECTION('ref_axis',(0.,-0.525379741809059,0.85086786688454));
#3986=DIRECTION('',(-1.,0.,0.));
#3987=DIRECTION('center_axis',(0.,0.,1.));
#3988=DIRECTION('ref_axis',(1.,0.,0.));
#3989=DIRECTION('',(-1.,9.01019857023267E-31,0.));
#3990=DIRECTION('center_axis',(0.,4.3841477367998E-16,-1.));
#3991=DIRECTION('ref_axis',(0.,1.,4.3841477367998E-16));
#3992=DIRECTION('',(1.,-9.01019857023267E-31,0.));
#3993=DIRECTION('center_axis',(0.,0.707106781186548,-0.707106781186548));
#3994=DIRECTION('ref_axis',(-1.,0.,0.));
#3995=DIRECTION('center_axis',(0.,0.707106781186547,0.707106781186548));
#3996=DIRECTION('ref_axis',(-1.,0.,0.));
#3997=DIRECTION('center_axis',(0.,0.707106781186548,-0.707106781186548));
#3998=DIRECTION('ref_axis',(-1.,0.,0.));
#3999=DIRECTION('center_axis',(0.,0.707106781186547,0.707106781186548));
#4000=DIRECTION('ref_axis',(-1.,0.,0.));
#4001=DIRECTION('center_axis',(0.,0.707106781186548,-0.707106781186548));
#4002=DIRECTION('ref_axis',(-1.,0.,0.));
#4003=DIRECTION('center_axis',(0.,0.707106781186547,0.707106781186548));
#4004=DIRECTION('ref_axis',(-1.,0.,0.));
#4005=DIRECTION('center_axis',(0.,0.707106781186548,-0.707106781186548));
#4006=DIRECTION('ref_axis',(-1.,0.,0.));
#4007=DIRECTION('center_axis',(0.,0.707106781186547,0.707106781186548));
#4008=DIRECTION('ref_axis',(-1.,0.,0.));
#4009=DIRECTION('center_axis',(0.,-0.707106781186547,-0.707106781186548));
#4010=DIRECTION('ref_axis',(1.,0.,0.));
#4011=DIRECTION('center_axis',(0.,-0.707106781186546,0.707106781186549));
#4012=DIRECTION('ref_axis',(1.,0.,0.));
#4013=DIRECTION('center_axis',(-6.37117250884884E-31,-0.707106781186546,
0.707106781186549));
#4014=DIRECTION('ref_axis',(1.,-9.01019857023267E-31,3.65180529852271E-47));
#4015=DIRECTION('center_axis',(-6.37117250884885E-31,-0.707106781186547,
-0.707106781186548));
#4016=DIRECTION('ref_axis',(1.,-9.01019857023266E-31,5.15319092140731E-47));
#4017=DIRECTION('center_axis',(-1.,0.,0.));
#4018=DIRECTION('ref_axis',(0.,0.,1.));
#4019=DIRECTION('center_axis',(1.,0.,0.));
#4020=DIRECTION('ref_axis',(0.,0.,-1.));
#4021=DIRECTION('center_axis',(1.,-9.01019857023267E-31,0.));
#4022=DIRECTION('ref_axis',(9.01019857023267E-31,1.,0.));
#4023=DIRECTION('center_axis',(1.,0.,0.));
#4024=DIRECTION('ref_axis',(0.,0.,-1.));
#4025=DIRECTION('center_axis',(-1.,9.01019857023267E-31,0.));
#4026=DIRECTION('ref_axis',(-9.01019857023267E-31,-1.,0.));
#4027=DIRECTION('center_axis',(-1.,0.,0.));
#4028=DIRECTION('ref_axis',(0.,0.,1.));
#4029=DIRECTION('center_axis',(-1.,0.,0.));
#4030=DIRECTION('ref_axis',(0.,0.,1.));
#4031=DIRECTION('center_axis',(-1.,0.,0.));
#4032=DIRECTION('ref_axis',(0.,0.,1.));
#4640=CARTESIAN_POINT('',(0.,0.,0.));
#4641=CARTESIAN_POINT('Origin',(180.,0.,240.));
#4642=CARTESIAN_POINT('',(180.,0.,235.));
#4643=CARTESIAN_POINT('',(180.,0.,215.000000000027));
#4644=CARTESIAN_POINT('',(180.,0.,240.));
#4645=CARTESIAN_POINT('',(176.58,0.,235.));
#4646=CARTESIAN_POINT('',(180.,0.,235.));
#4647=CARTESIAN_POINT('',(176.58,0.,215.000000000027));
#4648=CARTESIAN_POINT('',(176.58,0.,240.));
#4649=CARTESIAN_POINT('',(180.,0.,215.000000000027));
#4650=CARTESIAN_POINT('Origin',(3.42000000000001,0.,240.));
#4651=CARTESIAN_POINT('',(3.41999999999998,0.,235.));
#4652=CARTESIAN_POINT('',(3.42000000000001,0.,215.000000000027));
#4653=CARTESIAN_POINT('',(3.42000000000001,0.,240.));
#4654=CARTESIAN_POINT('',(0.,0.,235.));
#4655=CARTESIAN_POINT('',(3.41999999999998,0.,235.));
#4656=CARTESIAN_POINT('',(0.,0.,215.000000000027));
#4657=CARTESIAN_POINT('',(0.,0.,240.));
#4658=CARTESIAN_POINT('',(3.42000000000006,0.,215.000000000027));
#4659=CARTESIAN_POINT('Origin',(4.42000000000001,76.58,2.77555756156289E-14));
#4660=CARTESIAN_POINT('',(3.42000000000001,5.,0.));
#4661=CARTESIAN_POINT('',(3.42000000000001,33.5988232943213,0.));
#4662=CARTESIAN_POINT('',(3.42000000000001,0.,0.));
#4663=CARTESIAN_POINT('',(0.,5.,0.));
#4664=CARTESIAN_POINT('',(4.42000000000001,5.,2.77555756156289E-14));
#4665=CARTESIAN_POINT('',(0.,33.5988232943213,0.));
#4666=CARTESIAN_POINT('',(0.,0.,0.));
#4667=CARTESIAN_POINT('',(3.42000000000001,33.5988232943213,0.));
#4668=CARTESIAN_POINT('Origin',(175.58,76.58,240.));
#4669=CARTESIAN_POINT('',(176.58,33.5988232943213,240.));
#4670=CARTESIAN_POINT('',(176.58,5.,240.));
#4671=CARTESIAN_POINT('',(176.58,80.,240.));
#4672=CARTESIAN_POINT('',(180.,5.,240.));
#4673=CARTESIAN_POINT('',(175.58,5.,240.));
#4674=CARTESIAN_POINT('',(180.,33.5988232943213,240.));
#4675=CARTESIAN_POINT('',(180.,80.,240.));
#4676=CARTESIAN_POINT('',(176.58,33.5988232943213,240.));
#4677=CARTESIAN_POINT('Origin',(176.58,80.,240.));
#4678=CARTESIAN_POINT('',(176.58,33.5988232943213,2.77555756156289E-14));
#4679=CARTESIAN_POINT('',(176.58,5.,2.77555756156289E-14));
#4680=CARTESIAN_POINT('',(176.58,80.,2.77555756156289E-14));
#4681=CARTESIAN_POINT('',(176.58,0.,5.00000000000003));
#4682=CARTESIAN_POINT('Origin',(176.58,5.,5.00000000000002));
#4683=CARTESIAN_POINT('',(176.58,0.,24.9999999999819));
#4684=CARTESIAN_POINT('',(176.58,0.,240.));
#4685=CARTESIAN_POINT('',(176.58,5.00000000000003,29.9999999999819));
#4686=CARTESIAN_POINT('',(176.58,0.,24.9999999999819));
#4687=CARTESIAN_POINT('',(176.58,15.8272355779969,29.9999999999819));
#4688=CARTESIAN_POINT('',(176.58,80.0000000000001,29.999999999982));
#4689=CARTESIAN_POINT('',(176.58,27.1581715176779,43.0383298828501));
#4690=CARTESIAN_POINT('',(176.58,147.413588670352,181.414348191063));
#4691=CARTESIAN_POINT('',(176.58,27.1581715176779,83.0283770568992));
#4692=CARTESIAN_POINT('',(176.58,27.1581715176779,240.));
#4693=CARTESIAN_POINT('',(176.58,32.1581715176779,88.0283770568993));
#4694=CARTESIAN_POINT('',(176.58,27.1581715176779,83.0283770568992));
#4695=CARTESIAN_POINT('',(176.58,46.064656950061,88.0283770568993));
#4696=CARTESIAN_POINT('',(176.58,80.,88.0283770568993));
#4697=CARTESIAN_POINT('',(176.58,46.064656950061,93.0283770568993));
#4698=CARTESIAN_POINT('',(176.58,46.064656950061,240.));
#4699=CARTESIAN_POINT('',(176.58,25.0874391412115,93.0283770568993));
#4700=CARTESIAN_POINT('',(176.58,80.,93.0283770568993));
#4701=CARTESIAN_POINT('',(176.58,20.0874391412115,98.0283770568993));
#4702=CARTESIAN_POINT('',(176.58,25.0874391412115,93.0283770568993));
#4703=CARTESIAN_POINT('',(176.58,20.0874391412115,139.12816035213));
#4704=CARTESIAN_POINT('',(176.58,20.0874391412115,240.));
#4705=CARTESIAN_POINT('',(176.58,25.0874391412115,144.12816035213));
#4706=CARTESIAN_POINT('',(176.58,20.0874391412115,139.12816035213));
#4707=CARTESIAN_POINT('',(176.58,46.064656950061,144.12816035213));
#4708=CARTESIAN_POINT('',(176.58,80.,144.12816035213));
#4709=CARTESIAN_POINT('',(176.58,46.064656950061,149.12816035213));
#4710=CARTESIAN_POINT('',(176.58,46.064656950061,240.));
#4711=CARTESIAN_POINT('',(176.58,32.1581715176779,149.12816035213));
#4712=CARTESIAN_POINT('',(176.58,80.,149.12816035213));
#4713=CARTESIAN_POINT('',(176.58,27.1581715176779,154.12816035213));
#4714=CARTESIAN_POINT('',(176.58,32.1581715176779,149.12816035213));
#4715=CARTESIAN_POINT('',(176.58,27.1581715176779,191.649217650476));
#4716=CARTESIAN_POINT('',(176.58,27.1581715176779,240.));
#4717=CARTESIAN_POINT('',(176.58,15.8272355779969,210.000000000027));
#4718=CARTESIAN_POINT('',(176.58,20.1295883549968,203.032213771069));
#4719=CARTESIAN_POINT('',(176.58,5.00000000000003,210.000000000027));
#4720=CARTESIAN_POINT('',(176.58,80.,210.000000000027));
#4721=CARTESIAN_POINT('',(176.58,5.00000000000003,210.000000000027));
#4722=CARTESIAN_POINT('Origin',(176.58,5.,235.));
#4723=CARTESIAN_POINT('',(176.58,37.6255077137894,237.964087142109));
#4724=CARTESIAN_POINT('Origin',(176.58,33.5988232943213,235.));
#4725=CARTESIAN_POINT('',(176.58,75.58,186.403267432539));
#4726=CARTESIAN_POINT('',(176.58,51.5453007034368,219.054179684474));
#4727=CARTESIAN_POINT('',(176.58,75.58,53.5967325674605));
#4728=CARTESIAN_POINT('',(176.58,75.58,240.));
#4729=CARTESIAN_POINT('',(176.58,37.6255077137894,2.03591285789148));
#4730=CARTESIAN_POINT('',(176.58,166.125558428947,176.602019489803));
#4731=CARTESIAN_POINT('Origin',(176.58,33.5988232943213,5.00000000000002));
#4732=CARTESIAN_POINT('Origin',(180.,0.,240.));
#4733=CARTESIAN_POINT('',(180.,0.,5.00000000000003));
#4734=CARTESIAN_POINT('',(180.,0.,5.00000000000002));
#4735=CARTESIAN_POINT('',(180.,0.,24.999999999982));
#4736=CARTESIAN_POINT('',(180.,0.,240.));
#4737=CARTESIAN_POINT('',(176.58,0.,24.9999999999819));
#4738=CARTESIAN_POINT('Origin',(180.,80.,240.));
#4739=CARTESIAN_POINT('',(180.,5.,2.77555756156289E-14));
#4740=CARTESIAN_POINT('Origin',(180.,5.,5.00000000000002));
#4741=CARTESIAN_POINT('',(180.,33.5988232943213,2.77555756156289E-14));
#4742=CARTESIAN_POINT('',(180.,80.,2.77555756156289E-14));
#4743=CARTESIAN_POINT('',(180.,37.6255077137895,2.03591285789155));
#4744=CARTESIAN_POINT('Origin',(180.,33.5988232943213,5.00000000000002));
#4745=CARTESIAN_POINT('',(180.,75.58,53.5967325674606));
#4746=CARTESIAN_POINT('',(180.,32.4824320291808,-4.95090694006743));
#4747=CARTESIAN_POINT('',(180.,75.58,186.403267432539));
#4748=CARTESIAN_POINT('',(180.,75.58,240.));
#4749=CARTESIAN_POINT('',(180.,37.6255077137894,237.964087142108));
#4750=CARTESIAN_POINT('',(180.,32.4824320291808,244.950906940067));
#4751=CARTESIAN_POINT('Origin',(180.,33.5988232943213,235.));
#4752=CARTESIAN_POINT('Origin',(180.,5.,235.));
#4753=CARTESIAN_POINT('',(180.,5.00000000000003,210.000000000027));
#4754=CARTESIAN_POINT('',(180.,27.5000000000137,187.500000000014));
#4755=CARTESIAN_POINT('',(180.,15.8272355779969,210.000000000027));
#4756=CARTESIAN_POINT('',(180.,15.8272355779969,210.000000000027));
#4757=CARTESIAN_POINT('',(180.,27.1581715176779,191.649217650476));
#4758=CARTESIAN_POINT('',(180.,27.1581715176779,191.649217650476));
#4759=CARTESIAN_POINT('',(180.,27.1581715176779,154.12816035213));
#4760=CARTESIAN_POINT('',(180.,27.1581715176779,149.12816035213));
#4761=CARTESIAN_POINT('',(180.,32.1581715176779,149.12816035213));
#4762=CARTESIAN_POINT('',(180.,10.6431659349041,170.643165934904));
#4763=CARTESIAN_POINT('',(180.,46.064656950061,149.12816035213));
#4764=CARTESIAN_POINT('',(180.,46.064656950061,149.12816035213));
#4765=CARTESIAN_POINT('',(180.,46.064656950061,144.12816035213));
#4766=CARTESIAN_POINT('',(180.,46.064656950061,144.12816035213));
#4767=CARTESIAN_POINT('',(180.,25.0874391412115,144.12816035213));
#4768=CARTESIAN_POINT('',(180.,20.0874391412115,144.12816035213));
#4769=CARTESIAN_POINT('',(180.,20.0874391412115,139.12816035213));
#4770=CARTESIAN_POINT('',(180.,100.479639394541,219.520360605459));
#4771=CARTESIAN_POINT('',(180.,20.0874391412115,98.0283770568993));
#4772=CARTESIAN_POINT('',(180.,20.0874391412115,93.0283770568993));
#4773=CARTESIAN_POINT('',(180.,25.0874391412115,93.0283770568993));
#4774=CARTESIAN_POINT('',(180.,-20.9420919009446,139.057908099055));
#4775=CARTESIAN_POINT('',(180.,46.064656950061,93.0283770568993));
#4776=CARTESIAN_POINT('',(180.,46.064656950061,93.0283770568993));
#4777=CARTESIAN_POINT('',(180.,46.064656950061,88.0283770568993));
#4778=CARTESIAN_POINT('',(180.,46.064656950061,88.0283770568993));
#4779=CARTESIAN_POINT('',(180.,32.1581715176779,88.0283770568993));
#4780=CARTESIAN_POINT('',(180.,27.1581715176779,88.0283770568993));
#4781=CARTESIAN_POINT('',(180.,27.1581715176779,83.0283770568992));
#4782=CARTESIAN_POINT('',(180.,132.064897230389,187.935102769611));
#4783=CARTESIAN_POINT('',(180.,27.1581715176779,43.0383298828501));
#4784=CARTESIAN_POINT('',(180.,27.1581715176779,43.0383298828501));
#4785=CARTESIAN_POINT('',(180.,15.8272355779969,29.999999999982));
#4786=CARTESIAN_POINT('',(180.,15.8272355779969,29.999999999982));
#4787=CARTESIAN_POINT('',(180.,5.00000000000003,29.999999999982));
#4788=CARTESIAN_POINT('',(180.,15.8272355779969,29.999999999982));
#4789=CARTESIAN_POINT('',(180.,147.500000000009,172.499999999991));
#4790=CARTESIAN_POINT('Origin',(175.58,75.58,240.));
#4791=CARTESIAN_POINT('',(175.58,80.,180.398739130653));
#4792=CARTESIAN_POINT('Origin',(175.58,75.58,186.403267432539));
#4793=CARTESIAN_POINT('',(175.58,80.,59.6012608693474));
#4794=CARTESIAN_POINT('Origin',(175.579999999999,75.5799999999997,53.5967325674601));
#4795=CARTESIAN_POINT('',(175.58,80.,240.));
#4796=CARTESIAN_POINT('Origin',(0.,80.,240.));
#4797=CARTESIAN_POINT('',(4.41999999999998,80.,180.398739130653));
#4798=CARTESIAN_POINT('',(0.,80.,180.398739130653));
#4799=CARTESIAN_POINT('',(4.41999999999998,80.,59.6012608693474));
#4800=CARTESIAN_POINT('',(-5.55111512312578E-14,80.,59.6012608693474));
#4801=CARTESIAN_POINT('',(4.42000000000001,80.,240.));
#4802=CARTESIAN_POINT('Origin',(4.42000000000001,75.58,240.));
#4803=CARTESIAN_POINT('',(-5.55111512312578E-14,75.58,186.403267432539));
#4804=CARTESIAN_POINT('Origin',(4.42000000000044,75.5799999999996,186.40326743254));
#4805=CARTESIAN_POINT('',(0.,75.58,53.5967325674605));
#4806=CARTESIAN_POINT('Origin',(4.41999999999988,75.5800000000001,53.5967325674607));
#4807=CARTESIAN_POINT('',(0.,75.58,240.));
#4808=CARTESIAN_POINT('Origin',(0.,0.,240.));
#4809=CARTESIAN_POINT('',(0.,0.,5.));
#4810=CARTESIAN_POINT('Origin',(0.,5.,5.));
#4811=CARTESIAN_POINT('',(0.,0.,24.9999999999819));
#4812=CARTESIAN_POINT('',(0.,0.,240.));
#4813=CARTESIAN_POINT('',(0.,5.00000000000003,29.9999999999819));
#4814=CARTESIAN_POINT('',(0.,107.500000000009,132.499999999991));
#4815=CARTESIAN_POINT('',(0.,15.8272355779969,29.9999999999819));
#4816=CARTESIAN_POINT('',(0.,15.8272355779969,29.9999999999819));
#4817=CARTESIAN_POINT('',(-5.55111512312578E-14,27.1581715176779,43.0383298828501));
#4818=CARTESIAN_POINT('',(0.,15.8272355779969,29.9999999999819));
#4819=CARTESIAN_POINT('',(-5.55111512312578E-14,27.1581715176779,83.0283770568992));
#4820=CARTESIAN_POINT('',(-5.55111512312578E-14,27.1581715176779,43.0383298828501));
#4821=CARTESIAN_POINT('',(0.,32.1581715176779,88.0283770568993));
#4822=CARTESIAN_POINT('',(0.,92.0648972303893,147.935102769611));
#4823=CARTESIAN_POINT('',(0.,46.064656950061,88.0283770568993));
#4824=CARTESIAN_POINT('',(0.,27.1581715176779,88.0283770568993));
#4825=CARTESIAN_POINT('',(0.,46.064656950061,93.0283770568993));
#4826=CARTESIAN_POINT('',(0.,46.064656950061,88.0283770568993));
#4827=CARTESIAN_POINT('',(0.,25.0874391412115,93.0283770568993));
#4828=CARTESIAN_POINT('',(0.,46.064656950061,93.0283770568993));
#4829=CARTESIAN_POINT('',(-5.55111512312578E-14,20.0874391412115,98.0283770568993));
#4830=CARTESIAN_POINT('',(0.,-60.9420919009446,179.057908099055));
#4831=CARTESIAN_POINT('',(0.,20.0874391412115,139.12816035213));
#4832=CARTESIAN_POINT('',(0.,20.0874391412115,93.0283770568993));
#4833=CARTESIAN_POINT('',(0.,25.0874391412115,144.12816035213));
#4834=CARTESIAN_POINT('',(0.,60.4796393945406,179.520360605459));
#4835=CARTESIAN_POINT('',(0.,46.064656950061,144.12816035213));
#4836=CARTESIAN_POINT('',(0.,20.0874391412115,144.12816035213));
#4837=CARTESIAN_POINT('',(0.,46.064656950061,149.12816035213));
#4838=CARTESIAN_POINT('',(0.,46.064656950061,144.12816035213));
#4839=CARTESIAN_POINT('',(0.,32.1581715176779,149.12816035213));
#4840=CARTESIAN_POINT('',(0.,46.064656950061,149.12816035213));
#4841=CARTESIAN_POINT('',(-5.55111512312578E-14,27.1581715176779,154.12816035213));
#4842=CARTESIAN_POINT('',(-5.55111512312578E-14,-29.3568340650959,210.643165934904));
#4843=CARTESIAN_POINT('',(0.,27.1581715176779,191.649217650476));
#4844=CARTESIAN_POINT('',(0.,27.1581715176779,149.12816035213));
#4845=CARTESIAN_POINT('',(-5.55111512312578E-14,15.8272355779969,210.000000000027));
#4846=CARTESIAN_POINT('',(0.,27.1581715176779,191.649217650476));
#4847=CARTESIAN_POINT('',(-5.55111512312578E-14,5.00000000000003,210.000000000027));
#4848=CARTESIAN_POINT('',(-5.55111512312578E-14,15.8272355779969,210.000000000027));
#4849=CARTESIAN_POINT('',(0.,-12.4999999999863,227.500000000014));
#4850=CARTESIAN_POINT('',(0.,5.,240.));
#4851=CARTESIAN_POINT('Origin',(0.,5.,235.));
#4852=CARTESIAN_POINT('',(0.,33.5988232943213,240.));
#4853=CARTESIAN_POINT('',(0.,0.,240.));
#4854=CARTESIAN_POINT('',(0.,37.6255077137894,237.964087142108));
#4855=CARTESIAN_POINT('Origin',(0.,33.5988232943213,235.));
#4856=CARTESIAN_POINT('',(0.,32.4824320291808,244.950906940067));
#4857=CARTESIAN_POINT('',(0.,37.6255077137895,2.03591285789154));
#4858=CARTESIAN_POINT('',(-5.55111512312578E-14,32.4824320291808,-4.95090694006746));
#4859=CARTESIAN_POINT('Origin',(0.,33.5988232943213,5.));
#4860=CARTESIAN_POINT('Origin',(3.42000000000001,0.,240.));
#4861=CARTESIAN_POINT('',(3.41999999999998,0.,5.));
#4862=CARTESIAN_POINT('',(3.41999999999998,0.,5.));
#4863=CARTESIAN_POINT('',(3.42000000000001,0.,24.9999999999819));
#4864=CARTESIAN_POINT('',(3.42000000000001,0.,240.));
#4865=CARTESIAN_POINT('',(0.,0.,24.9999999999819));
#4866=CARTESIAN_POINT('Origin',(3.42000000000001,0.,240.));
#4867=CARTESIAN_POINT('Origin',(3.41999999999998,5.,5.));
#4868=CARTESIAN_POINT('',(3.42000000000001,37.6255077137895,2.03591285789145));
#4869=CARTESIAN_POINT('Origin',(3.42000000000001,33.5988232943213,5.));
#4870=CARTESIAN_POINT('',(3.42000000000001,75.58,53.5967325674606));
#4871=CARTESIAN_POINT('',(3.41999999999995,138.010958153706,138.408600247967));
#4872=CARTESIAN_POINT('',(3.41999999999995,75.58,186.403267432539));
#4873=CARTESIAN_POINT('',(3.42000000000001,75.58,240.));
#4874=CARTESIAN_POINT('',(3.42000000000001,37.6255077137895,237.964087142109));
#4875=CARTESIAN_POINT('',(3.41999999999995,23.430700428196,257.247598926311));
#4876=CARTESIAN_POINT('',(3.42000000000001,33.5988232943213,240.));
#4877=CARTESIAN_POINT('Origin',(3.42000000000001,33.5988232943213,235.));
#4878=CARTESIAN_POINT('',(3.42000000000001,5.,240.));
#4879=CARTESIAN_POINT('',(3.42000000000001,0.,240.));
#4880=CARTESIAN_POINT('Origin',(3.41999999999998,5.,235.));
#4881=CARTESIAN_POINT('',(3.41999999999995,5.00000000000003,210.000000000027));
#4882=CARTESIAN_POINT('',(3.41999999999995,5.00000000000003,210.000000000027));
#4883=CARTESIAN_POINT('',(3.42000000000001,15.8272355779969,210.000000000027));
#4884=CARTESIAN_POINT('',(3.41999999999995,0.,210.000000000027));
#4885=CARTESIAN_POINT('',(3.42000000000006,27.1581715176779,191.649217650476));
#4886=CARTESIAN_POINT('',(3.42000000000001,-1.95232149327149,238.794512988463));
#4887=CARTESIAN_POINT('',(3.41999999999995,27.1581715176779,154.12816035213));
#4888=CARTESIAN_POINT('',(3.42000000000001,27.1581715176779,240.));
#4889=CARTESIAN_POINT('',(3.42000000000001,32.1581715176779,149.12816035213));
#4890=CARTESIAN_POINT('',(3.42000000000001,32.1581715176779,149.12816035213));
#4891=CARTESIAN_POINT('',(3.42000000000006,46.064656950061,149.12816035213));
#4892=CARTESIAN_POINT('',(3.42000000000001,0.,149.12816035213));
#4893=CARTESIAN_POINT('',(3.42000000000006,46.064656950061,144.12816035213));
#4894=CARTESIAN_POINT('',(3.42000000000001,46.064656950061,240.));
#4895=CARTESIAN_POINT('',(3.42000000000001,25.0874391412115,144.12816035213));
#4896=CARTESIAN_POINT('',(3.42000000000001,0.,144.12816035213));
#4897=CARTESIAN_POINT('',(3.41999999999998,20.0874391412115,139.12816035213));
#4898=CARTESIAN_POINT('',(3.41999999999998,20.0874391412115,139.12816035213));
#4899=CARTESIAN_POINT('',(3.41999999999995,20.0874391412115,98.0283770568993));
#4900=CARTESIAN_POINT('',(3.42000000000001,20.0874391412115,240.));
#4901=CARTESIAN_POINT('',(3.41999999999998,25.0874391412115,93.0283770568993));
#4902=CARTESIAN_POINT('',(3.42000000000001,25.0874391412115,93.0283770568993));
#4903=CARTESIAN_POINT('',(3.42000000000006,46.064656950061,93.0283770568993));
#4904=CARTESIAN_POINT('',(3.41999999999998,0.,93.0283770568993));
#4905=CARTESIAN_POINT('',(3.42000000000006,46.064656950061,88.0283770568993));
#4906=CARTESIAN_POINT('',(3.42000000000001,46.064656950061,240.));
#4907=CARTESIAN_POINT('',(3.42000000000001,32.1581715176779,88.0283770568993));
#4908=CARTESIAN_POINT('',(3.42000000000001,0.,88.0283770568993));
#4909=CARTESIAN_POINT('',(3.41999999999995,27.1581715176779,83.0283770568992));
#4910=CARTESIAN_POINT('',(3.41999999999995,27.1581715176779,83.0283770568992));
#4911=CARTESIAN_POINT('',(3.42000000000001,27.1581715176779,43.0383298828501));
#4912=CARTESIAN_POINT('',(3.42000000000001,27.1581715176779,240.));
#4913=CARTESIAN_POINT('',(3.42000000000006,15.8272355779969,29.9999999999819));
#4914=CARTESIAN_POINT('',(3.42000000000001,112.991281499218,141.805140389003));
#4915=CARTESIAN_POINT('',(3.42000000000001,5.00000000000003,29.9999999999819));
#4916=CARTESIAN_POINT('',(3.42000000000001,9.0205620750794E-14,29.9999999999819));
#4917=CARTESIAN_POINT('',(3.42000000000001,0.,24.9999999999819));
#4918=CARTESIAN_POINT('Origin',(4.42000000000001,75.58,240.));
#4919=CARTESIAN_POINT('',(4.42000000000001,76.58,185.044776866502));
#4920=CARTESIAN_POINT('',(4.42000000000001,76.58,54.9552231334983));
#4921=CARTESIAN_POINT('',(4.42000000000001,76.58,240.));
#4922=CARTESIAN_POINT('Origin',(4.42000000000056,75.5799999999996,186.40326743254));
#4923=CARTESIAN_POINT('Origin',(4.41999999999978,75.5800000000002,53.5967325674609));
#4924=CARTESIAN_POINT('Origin',(0.,76.58,240.));
#4925=CARTESIAN_POINT('',(175.58,76.58,185.044776866502));
#4926=CARTESIAN_POINT('',(175.58,76.58,54.9552231334984));
#4927=CARTESIAN_POINT('',(175.58,76.58,240.));
#4928=CARTESIAN_POINT('',(0.,76.58,185.044776866502));
#4929=CARTESIAN_POINT('',(0.,76.58,54.9552231334983));
#4930=CARTESIAN_POINT('Origin',(175.58,75.58,240.));
#4931=CARTESIAN_POINT('Origin',(175.580000000001,75.5800000000019,186.403267432537));
#4932=CARTESIAN_POINT('Origin',(175.58,75.5799999999998,53.5967325674603));
#4933=CARTESIAN_POINT('Origin',(175.58,75.58,240.));
#4934=CARTESIAN_POINT('',(175.58,5.,240.));
#4935=CARTESIAN_POINT('',(0.,33.5988232943213,240.));
#4936=CARTESIAN_POINT('Origin',(175.58,75.58,2.77555756156289E-14));
#4937=CARTESIAN_POINT('',(176.58,5.,2.77555756156289E-14));
#4938=CARTESIAN_POINT('',(175.58,33.5988232943213,2.77555756156289E-14));
#4939=CARTESIAN_POINT('Origin',(180.,32.4824320291808,-4.95090694006743));
#4940=CARTESIAN_POINT('',(0.,37.6255077137895,2.03591285789154));
#4941=CARTESIAN_POINT('',(180.,37.6255077137895,2.03591285789155));
#4942=CARTESIAN_POINT('Origin',(180.,32.4824320291808,244.950906940067));
#4943=CARTESIAN_POINT('',(180.,37.6255077137894,237.964087142108));
#4944=CARTESIAN_POINT('',(3.42000000000001,37.6255077137894,237.964087142109));
#4945=CARTESIAN_POINT('Origin',(180.,15.8272355779969,29.999999999982));
#4946=CARTESIAN_POINT('',(3.42000000000001,5.00000000000003,29.9999999999819));
#4947=CARTESIAN_POINT('',(180.,15.8272355779969,29.999999999982));
#4948=CARTESIAN_POINT('Origin',(180.,15.8272355779969,210.000000000027));
#4949=CARTESIAN_POINT('',(-5.55111512312578E-14,5.00000000000003,210.000000000027));
#4950=CARTESIAN_POINT('',(180.,15.8272355779969,210.000000000027));
#4951=CARTESIAN_POINT('Origin',(180.,27.1581715176779,191.649217650476));
#4952=CARTESIAN_POINT('',(180.,27.1581715176779,191.649217650476));
#4953=CARTESIAN_POINT('Origin',(180.,27.1581715176779,149.12816035213));
#4954=CARTESIAN_POINT('',(180.,27.1581715176779,154.12816035213));
#4955=CARTESIAN_POINT('Origin',(180.,46.064656950061,149.12816035213));
#4956=CARTESIAN_POINT('',(180.,32.1581715176779,149.12816035213));
#4957=CARTESIAN_POINT('',(180.,46.064656950061,149.12816035213));
#4958=CARTESIAN_POINT('Origin',(180.,46.064656950061,144.12816035213));
#4959=CARTESIAN_POINT('',(180.,46.064656950061,144.12816035213));
#4960=CARTESIAN_POINT('Origin',(180.,20.0874391412115,144.12816035213));
#4961=CARTESIAN_POINT('',(180.,25.0874391412115,144.12816035213));
#4962=CARTESIAN_POINT('Origin',(180.,20.0874391412115,93.0283770568993));
#4963=CARTESIAN_POINT('',(180.,20.0874391412115,98.0283770568993));
#4964=CARTESIAN_POINT('',(180.,20.0874391412115,139.12816035213));
#4965=CARTESIAN_POINT('Origin',(180.,46.064656950061,93.0283770568993));
#4966=CARTESIAN_POINT('',(180.,25.0874391412115,93.0283770568993));
#4967=CARTESIAN_POINT('',(180.,46.064656950061,93.0283770568993));
#4968=CARTESIAN_POINT('Origin',(180.,46.064656950061,88.0283770568993));
#4969=CARTESIAN_POINT('',(180.,46.064656950061,88.0283770568993));
#4970=CARTESIAN_POINT('Origin',(180.,27.1581715176779,88.0283770568993));
#4971=CARTESIAN_POINT('',(180.,32.1581715176779,88.0283770568993));
#4972=CARTESIAN_POINT('Origin',(180.,27.1581715176779,43.0383298828501));
#4973=CARTESIAN_POINT('',(180.,27.1581715176779,83.0283770568992));
#4974=CARTESIAN_POINT('',(180.,27.1581715176779,43.0383298828501));
#4975=CARTESIAN_POINT('Origin',(180.,15.8272355779969,29.999999999982));
#4976=CARTESIAN_POINT('Origin',(180.,15.8272355779969,29.999999999982));
#4977=CARTESIAN_POINT('',(180.,15.8272355779969,29.999999999982));
#4978=CARTESIAN_POINT('',(180.,27.1581715176779,43.0383298828501));
#4979=CARTESIAN_POINT('Origin',(180.,27.1581715176779,43.0383298828501));
#4980=CARTESIAN_POINT('',(180.,27.1581715176779,83.0283770568992));
#4981=CARTESIAN_POINT('Origin',(180.,27.1581715176779,88.0283770568993));
#4982=CARTESIAN_POINT('',(180.,32.1581715176779,88.0283770568993));
#4983=CARTESIAN_POINT('',(180.,46.064656950061,88.0283770568993));
#4984=CARTESIAN_POINT('Origin',(180.,46.064656950061,88.0283770568993));
#4985=CARTESIAN_POINT('',(180.,46.064656950061,93.0283770568993));
#4986=CARTESIAN_POINT('Origin',(180.,46.064656950061,93.0283770568993));
#4987=CARTESIAN_POINT('',(180.,25.0874391412115,93.0283770568993));
#4988=CARTESIAN_POINT('Origin',(180.,20.0874391412115,93.0283770568993));
#4989=CARTESIAN_POINT('',(180.,20.0874391412115,98.0283770568993));
#4990=CARTESIAN_POINT('',(180.,20.0874391412115,139.12816035213));
#4991=CARTESIAN_POINT('Origin',(180.,20.0874391412115,144.12816035213));
#4992=CARTESIAN_POINT('',(180.,25.0874391412115,144.12816035213));
#4993=CARTESIAN_POINT('',(180.,46.064656950061,144.12816035213));
#4994=CARTESIAN_POINT('Origin',(180.,46.064656950061,144.12816035213));
#4995=CARTESIAN_POINT('',(180.,46.064656950061,149.12816035213));
#4996=CARTESIAN_POINT('Origin',(180.,46.064656950061,149.12816035213));
#4997=CARTESIAN_POINT('',(180.,32.1581715176779,149.12816035213));
#4998=CARTESIAN_POINT('Origin',(180.,27.1581715176779,149.12816035213));
#4999=CARTESIAN_POINT('',(180.,27.1581715176779,154.12816035213));
#5000=CARTESIAN_POINT('',(180.,27.1581715176779,191.649217650476));
#5001=CARTESIAN_POINT('Origin',(180.,27.1581715176779,191.649217650476));
#5002=CARTESIAN_POINT('',(180.,15.8272355779969,210.000000000027));
#5003=CARTESIAN_POINT('Origin',(180.,15.8272355779969,210.000000000027));
#5004=CARTESIAN_POINT('',(176.58,5.00000000000003,210.000000000027));
#5005=CARTESIAN_POINT('Origin',(180.,15.8272355779969,29.999999999982));
#5006=CARTESIAN_POINT('',(180.,5.00000000000003,29.999999999982));
#5007=CARTESIAN_POINT('Origin',(180.,20.0874391412115,139.12816035213));
#5008=CARTESIAN_POINT('Origin',(180.,25.0874391412115,93.0283770568993));
#5009=CARTESIAN_POINT('Origin',(180.,27.1581715176779,83.0283770568992));
#5010=CARTESIAN_POINT('Origin',(180.,32.1581715176779,149.12816035213));
#5011=CARTESIAN_POINT('Origin',(180.,20.0874391412115,139.12816035213));
#5012=CARTESIAN_POINT('Origin',(180.,32.1581715176779,149.12816035213));
#5013=CARTESIAN_POINT('Origin',(180.,27.1581715176779,83.0283770568992));
#5014=CARTESIAN_POINT('Origin',(180.,25.0874391412115,93.0283770568993));
#5015=CARTESIAN_POINT('Origin',(180.,5.00000000000003,210.000000000027));
#5016=CARTESIAN_POINT('Origin',(3.42000000000001,0.,24.9999999999819));
#5017=CARTESIAN_POINT('Origin',(180.,0.,24.999999999982));
#5018=CARTESIAN_POINT('Origin',(180.,5.00000000000003,210.000000000027));
#5019=CARTESIAN_POINT('Origin',(4.41999999999998,5.,5.00000000000003));
#5020=CARTESIAN_POINT('Origin',(180.,33.5988232943213,5.00000000000002));
#5021=CARTESIAN_POINT('Origin',(175.58,5.,5.00000000000003));
#5022=CARTESIAN_POINT('Origin',(175.58,33.5988232943213,5.00000000000003));
#5023=CARTESIAN_POINT('Origin',(180.,5.,235.));
#5024=CARTESIAN_POINT('Origin',(180.,33.5988232943213,235.));
#5025=CARTESIAN_POINT('Origin',(3.41999999999998,5.,235.));
#5026=CARTESIAN_POINT('Origin',(180.,33.5988232943213,235.));
#5585=UNCERTAINTY_MEASURE_WITH_UNIT(LENGTH_MEASURE(0.01),#5600,
'DISTANCE_ACCURACY_VALUE',
'Maximum model space distance between geometric entities at asserted c
onnectivities');
#5591=UNCERTAINTY_MEASURE_WITH_UNIT(LENGTH_MEASURE(0.01),#5600,
'DISTANCE_ACCURACY_VALUE',
'Maximum model space distance between geometric entities at asserted c
onnectivities');
#5593=(
GEOMETRIC_REPRESENTATION_CONTEXT(3)
GLOBAL_UNCERTAINTY_ASSIGNED_CONTEXT((#5585))
GLOBAL_UNIT_ASSIGNED_CONTEXT((#5600,#5602,#5603))
REPRESENTATION_CONTEXT('','3D')
);
#5599=(
GEOMETRIC_REPRESENTATION_CONTEXT(3)
GLOBAL_UNCERTAINTY_ASSIGNED_CONTEXT((#5591))
GLOBAL_UNIT_ASSIGNED_CONTEXT((#5600,#5602,#5603))
REPRESENTATION_CONTEXT('','3D')
);
#5600=(
LENGTH_UNIT()
NAMED_UNIT(*)
SI_UNIT(.MILLI.,.METRE.)
);
#5602=(
NAMED_UNIT(*)
PLANE_ANGLE_UNIT()
SI_UNIT($,.RADIAN.)
);
#5603=(
NAMED_UNIT(*)
SI_UNIT($,.STERADIAN.)
SOLID_ANGLE_UNIT()
);
#5605=SHAPE_DEFINITION_REPRESENTATION(#5612,#5641);
#5612=PRODUCT_DEFINITION_SHAPE('',$,#5649);
#5641=SHAPE_REPRESENTATION('',(#3381),#5593);
#5647=PRODUCT_DEFINITION_CONTEXT('part definition',#5670,'design');
#5649=PRODUCT_DEFINITION('Gauge','Gauge',#5656,#5647);
#5656=PRODUCT_DEFINITION_FORMATION('',$,#5673);
#5670=APPLICATION_CONTEXT(
'Core Data for Automotive Mechanical Design Process');
#5671=PRODUCT_CONTEXT('part definition',#5670,'mechanical');
#5673=PRODUCT('Gauge','Gauge',$,(#5671));
#5680=PRESENTATION_STYLE_ASSIGNMENT((#5683));
#5683=SURFACE_STYLE_USAGE(.BOTH.,#5686);
#5686=SURFACE_SIDE_STYLE('',(#5689));
#5689=SURFACE_STYLE_FILL_AREA(#5692);
#5692=FILL_AREA_STYLE('Opaque(97,158,199)',(#5695));
#5695=FILL_AREA_STYLE_COLOUR('Opaque(97,158,199)',#5698);
#5698=COLOUR_RGB('Opaque(97,158,199)',0.380392156862745,0.619607843137255,
0.780392156862745);
ENDSEC;
END-ISO-10303-21;
